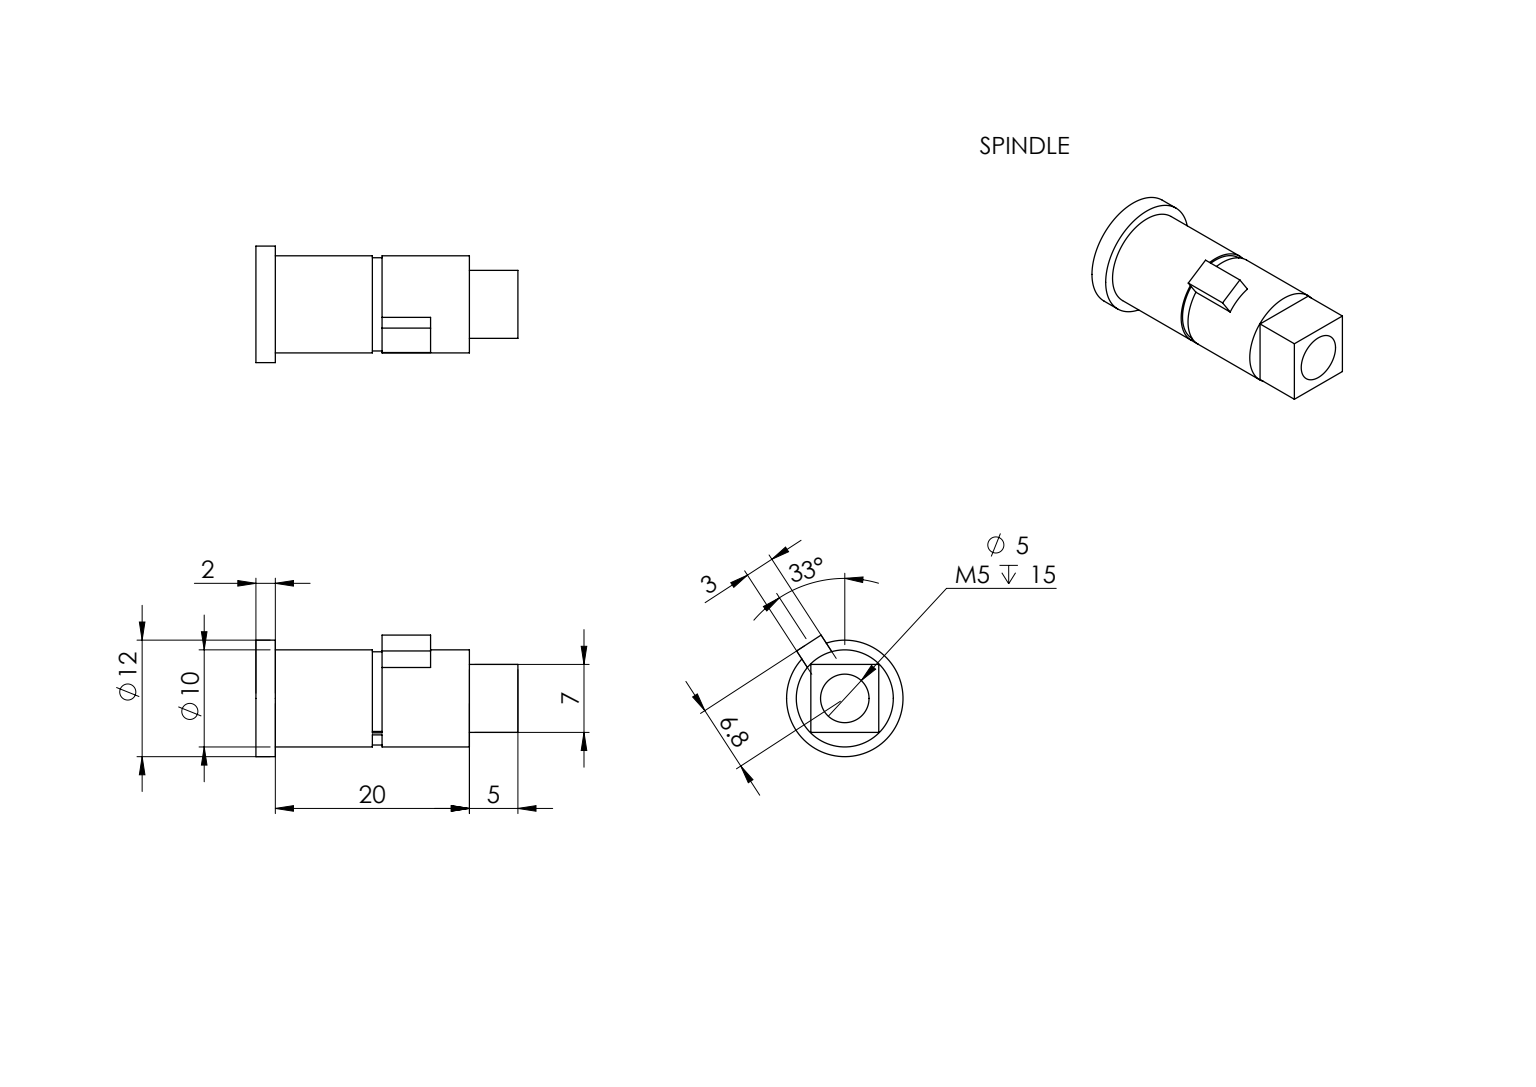
ISO-10303-21;
HEADER;
FILE_DESCRIPTION (('STEP AP214'),
    '1' );
FILE_NAME ('spindle.step',
    '2026-10-27T08:02:39',
    ( '' ),
    ( '' ),
    'SwSTEP 2.0',
    'SolidWorks 2026',
    '' );
FILE_SCHEMA (( 'AUTOMOTIVE_DESIGN' ));
ENDSEC;

DATA;
#32=DIRECTION ( 'NONE',  ( 1.000000000000000000, -0.000000000000000000, 0.000000000000000000 ) ) ;
#36=AXIS2_PLACEMENT_3D ( 'NONE', #6295, #7112, #8236 ) ;
#46=DIRECTION ( 'NONE',  ( 0.000000000000000000, 0.000000000000000000, -1.000000000000000000 ) ) ;
#52=ORIENTED_EDGE ( 'NONE', *, *, #6778, .T. ) ;
#65=DIRECTION ( 'NONE',  ( 0.000000000000000000, 0.6828850436591804574, 0.7305258497456468270 ) ) ;
#79=DIRECTION ( 'NONE',  ( -1.000000000000000000, 0.000000000000000000, 0.000000000000000000 ) ) ;
#82=EDGE_LOOP ( 'NONE', ( #2699, #3221, #1279, #723 ) ) ;
#84=CARTESIAN_POINT ( 'NONE',  ( 36.00000000000000711, -3.606021680338235225, -38.83193945118931367 ) ) ;
#99=DIRECTION ( 'NONE',  ( 0.000000000000000000, 0.6828850436591804574, 0.7305258497456468270 ) ) ;
#101=EDGE_LOOP ( 'NONE', ( #11163, #3779, #6204, #11294 ) ) ;
#116=ORIENTED_EDGE ( 'NONE', *, *, #4223, .F. ) ;
#145=DIRECTION ( 'NONE',  ( 0.000000000000000000, 0.000000000000000000, -1.000000000000000000 ) ) ;
#166=EDGE_LOOP ( 'NONE', ( #4533, #1972 ) ) ;
#181=CYLINDRICAL_SURFACE ( 'NONE', #468, 5.000000000000004441 ) ;
#194=CARTESIAN_POINT ( 'NONE',  ( 51.00000000000000000, -3.499999999999998668, -45.49999999999998579 ) ) ;
#212=CARTESIAN_POINT ( 'NONE',  ( 0.000000000000000000, 0.000000000000000000, 0.000000000000000000 ) ) ;
#214=VERTEX_POINT ( 'NONE', #5344 ) ;
#240=AXIS2_PLACEMENT_3D ( 'NONE', #7909, #5962, #9852 ) ;
#243=CONICAL_SURFACE ( 'NONE', #4238, 2.500000000000002220, 1.029744260000000189 ) ;
#251=LINE ( 'NONE', #9999, #3639 ) ;
#274=AXIS2_PLACEMENT_3D ( 'NONE', #11157, #11099, #1724 ) ;
#281=ORIENTED_EDGE ( 'NONE', *, *, #4388, .F. ) ;
#284=CIRCLE ( 'NONE', #2474, 4.800000000000000711 ) ;
#287=ADVANCED_FACE ( 'NONE', ( #2841 ), #4660, .F. ) ;
#293=PLANE ( 'NONE',  #3827 ) ;
#330=PRODUCT ( 'spindle', 'spindle', '', ( #11158 ) ) ;
#346=ORIENTED_EDGE ( 'NONE', *, *, #9732, .F. ) ;
#349=MANIFOLD_SOLID_BREP ( 'AdvancedHole1', #10962 ) ;
#352=EDGE_CURVE ( 'NONE', #7364, #3914, #3801, .T. ) ;
#364=CARTESIAN_POINT ( 'NONE',  ( 42.00000000000000000, 3.183245106666225510, -38.14423151746819229 ) ) ;
#375=DIRECTION ( 'NONE',  ( 0.000000000000000000, 0.000000000000000000, 1.000000000000000000 ) ) ;
#427=DIRECTION ( 'NONE',  ( 1.000000000000000000, -0.000000000000000000, -0.000000000000000000 ) ) ;
#441=CARTESIAN_POINT ( 'NONE',  ( 46.00000000000000000, 3.500000000000001332, -38.49999999999998579 ) ) ;
#458=CARTESIAN_POINT ( 'NONE',  ( 46.00000000000000000, 6.123233995736773185E-16, -46.99999999999999289 ) ) ;
#468=AXIS2_PLACEMENT_3D ( 'NONE', #2246, #10558, #8702 ) ;
#494=( LENGTH_UNIT ( ) NAMED_UNIT ( * ) SI_UNIT ( .MILLI., .METRE. ) );
#520=DIRECTION ( 'NONE',  ( -1.000000000000000000, -0.000000000000000000, -0.000000000000000000 ) ) ;
#524=ORIENTED_EDGE ( 'NONE', *, *, #1950, .F. ) ;
#553=ORIENTED_EDGE ( 'NONE', *, *, #10197, .F. ) ;
#554=ORIENTED_EDGE ( 'NONE', *, *, #10262, .T. ) ;
#565=ADVANCED_FACE ( 'NONE', ( #4744 ), #6885, .T. ) ;
#574=CARTESIAN_POINT ( 'NONE',  ( 51.00000000000000000, -3.499999999999998668, -38.49999999999998579 ) ) ;
#586=CARTESIAN_POINT ( 'NONE',  ( 42.00000000000000000, 4.817162211711309538, -40.66024322130446222 ) ) ;
#593=EDGE_CURVE ( 'NONE', #6667, #1161, #5812, .T. ) ;
#608=VECTOR ( 'NONE', #3199, 1000.000000000000000 ) ;
#615=AXIS2_PLACEMENT_3D ( 'NONE', #2148, #3107, #7677 ) ;
#627=ORIENTED_EDGE ( 'NONE', *, *, #11894, .F. ) ;
#631=COLOUR_RGB ( '',0.8941176470588234615, 0.8941176470588234615, 0.8941176470588234615 ) ;
#632=AXIS2_PLACEMENT_3D ( 'NONE', #3534, #3664, #4664 ) ;
#638=ADVANCED_FACE ( 'NONE', ( #2934 ), #10626, .T. ) ;
#654=AXIS2_PLACEMENT_3D ( 'NONE', #12142, #12213, #1855 ) ;
#659=PLANE ( 'NONE',  #632 ) ;
#679=ORIENTED_EDGE ( 'NONE', *, *, #2867, .F. ) ;
#681=VERTEX_POINT ( 'NONE', #9507 ) ;
#698=DIRECTION ( 'NONE',  ( 1.000000000000000000, 0.000000000000000000, 0.000000000000000000 ) ) ;
#716=DIRECTION ( 'NONE',  ( -1.000000000000000000, -0.000000000000000000, -0.000000000000000000 ) ) ;
#723=ORIENTED_EDGE ( 'NONE', *, *, #8714, .T. ) ;
#750=DIRECTION ( 'NONE',  ( 0.000000000000000000, 0.000000000000000000, 1.000000000000000000 ) ) ;
#777=VERTEX_POINT ( 'NONE', #5243 ) ;
#787=MECHANICAL_DESIGN_GEOMETRIC_PRESENTATION_REPRESENTATION('',(#4384),#9194);
#812=CARTESIAN_POINT ( 'NONE',  ( 36.00000000000000711, 1.456773409934505593E-31, -36.99999999999998579 ) ) ;
#822=EDGE_CURVE ( 'NONE', #4760, #6667, #10739, .T. ) ;
#832=AXIS2_PLACEMENT_3D ( 'NONE', #4718, #6732, #8723 ) ;
#853=AXIS2_PLACEMENT_3D ( 'NONE', #10883, #7084, #7954 ) ;
#861=AXIS2_PLACEMENT_3D ( 'NONE', #6268, #3378, #6379 ) ;
#863=VERTEX_POINT ( 'NONE', #1425 ) ;
#877=AXIS2_PLACEMENT_3D ( 'NONE', #8794, #2853, #1099 ) ;
#878=SURFACE_STYLE_USAGE ( .BOTH. , #7454 ) ;
#893=DIRECTION ( 'NONE',  ( 0.000000000000000000, 0.000000000000000000, 1.000000000000000000 ) ) ;
#924=ORIENTED_EDGE ( 'NONE', *, *, #6368, .T. ) ;
#951=ADVANCED_FACE ( 'NONE', ( #2674 ), #3495, .T. ) ;
#974=DIRECTION ( 'NONE',  ( 1.000000000000000000, -0.000000000000000000, -0.000000000000000000 ) ) ;
#991=CIRCLE ( 'NONE', #11951, 6.000000000000005329 ) ;
#1006=AXIS2_PLACEMENT_3D ( 'NONE', #1909, #9667, #145 ) ;
#1007=LINE ( 'NONE', #5641, #2212 ) ;
#1068=DIRECTION ( 'NONE',  ( -1.000000000000000000, 0.000000000000000000, 0.000000000000000000 ) ) ;
#1070=CARTESIAN_POINT ( 'NONE',  ( 24.00000000000000000, 0.000000000000000000, -48.00000000000000000 ) ) ;
#1099=DIRECTION ( 'NONE',  ( 0.000000000000000000, 0.000000000000000000, -1.000000000000000000 ) ) ;
#1112=EDGE_CURVE ( 'NONE', #1842, #1155, #6743, .T. ) ;
#1148=DIRECTION ( 'NONE',  ( -1.000000000000000000, -0.000000000000000000, -0.000000000000000000 ) ) ;
#1155=VERTEX_POINT ( 'NONE', #7617 ) ;
#1160=ORIENTED_EDGE ( 'NONE', *, *, #3799, .T. ) ;
#1161=VERTEX_POINT ( 'NONE', #7111 ) ;
#1181=FACE_OUTER_BOUND ( 'NONE', #4103, .T. ) ;
#1196=EDGE_LOOP ( 'NONE', ( #10186, #2981, #11180, #8301 ) ) ;
#1261=CARTESIAN_POINT ( 'NONE',  ( 37.00000000000000711, 1.456773409934505593E-31, -41.99999999999998579 ) ) ;
#1279=ORIENTED_EDGE ( 'NONE', *, *, #11894, .T. ) ;
#1283=ORIENTED_EDGE ( 'NONE', *, *, #11655, .F. ) ;
#1309=CARTESIAN_POINT ( 'NONE',  ( 51.00000000000000000, 0.000000000000000000, -41.99999999999999289 ) ) ;
#1313=DIRECTION ( 'NONE',  ( 0.000000000000000000, 0.000000000000000000, 1.000000000000000000 ) ) ;
#1318=LINE ( 'NONE', #7616, #9969 ) ;
#1362=EDGE_LOOP ( 'NONE', ( #3805, #3426, #3636, #11704 ) ) ;
#1369=DIRECTION ( 'NONE',  ( 1.000000000000000000, -0.000000000000000000, -0.000000000000000000 ) ) ;
#1373=EDGE_LOOP ( 'NONE', ( #11318, #8359, #9664, #4705 ) ) ;
#1425=CARTESIAN_POINT ( 'NONE',  ( 36.00000000000000711, 3.277848209564065307, -38.49347592122088457 ) ) ;
#1438=ORIENTED_EDGE ( 'NONE', *, *, #6782, .T. ) ;
#1457=CIRCLE ( 'NONE', #654, 6.000000000000005329 ) ;
#1472=ORIENTED_EDGE ( 'NONE', *, *, #11211, .F. ) ;
#1480=DIRECTION ( 'NONE',  ( 0.000000000000000000, -0.5446390350150287496, 0.8386705679454229401 ) ) ;
#1481=ORIENTED_EDGE ( 'NONE', *, *, #6301, .T. ) ;
#1513=EDGE_LOOP ( 'NONE', ( #1666, #2104, #8806 ) ) ;
#1525=DIRECTION ( 'NONE',  ( -0.000000000000000000, 0.8386705679454227180, 0.5446390350150290827 ) ) ;
#1533=DIRECTION ( 'NONE',  ( -1.000000000000000000, 0.000000000000000000, 0.000000000000000000 ) ) ;
#1545=ORIENTED_EDGE ( 'NONE', *, *, #3493, .F. ) ;
#1566=ORIENTED_EDGE ( 'NONE', *, *, #6391, .F. ) ;
#1586=AXIS2_PLACEMENT_3D ( 'NONE', #6572, #7575, #9517 ) ;
#1636=DIRECTION ( 'NONE',  ( -1.000000000000000000, 0.000000000000000000, 0.000000000000000000 ) ) ;
#1640=CIRCLE ( 'NONE', #240, 2.500000000000002220 ) ;
#1658=EDGE_CURVE ( 'NONE', #4309, #2267, #8104, .T. ) ;
#1659=AXIS2_PLACEMENT_3D ( 'NONE', #4254, #2260, #4307 ) ;
#1666=ORIENTED_EDGE ( 'NONE', *, *, #1679, .F. ) ;
#1679=EDGE_CURVE ( 'NONE', #11493, #5674, #6035, .T. ) ;
#1698=CARTESIAN_POINT ( 'NONE',  ( 37.00000000000000711, 1.456773409934505593E-31, -41.99999999999998579 ) ) ;
#1711=ORIENTED_EDGE ( 'NONE', *, *, #7878, .F. ) ;
#1712=EDGE_CURVE ( 'NONE', #11907, #4096, #9726, .T. ) ;
#1724=DIRECTION ( 'NONE',  ( 0.000000000000000000, 0.000000000000000000, 1.000000000000000000 ) ) ;
#1750=PRESENTATION_STYLE_ASSIGNMENT (( #878 ) ) ;
#1767=UNCERTAINTY_MEASURE_WITH_UNIT (LENGTH_MEASURE( 1.000000000000000082E-05 ), #3696, 'distance_accuracy_value', 'NONE');
#1792=ORIENTED_EDGE ( 'NONE', *, *, #1712, .F. ) ;
#1814=LINE ( 'NONE', #7453, #11245 ) ;
#1831=DIRECTION ( 'NONE',  ( -1.000000000000000000, 0.000000000000000000, 0.000000000000000000 ) ) ;
#1842=VERTEX_POINT ( 'NONE', #9101 ) ;
#1843=CIRCLE ( 'NONE', #11015, 5.000000000000004441 ) ;
#1855=DIRECTION ( 'NONE',  ( 0.000000000000000000, 0.000000000000000000, 1.000000000000000000 ) ) ;
#1856=ORIENTED_EDGE ( 'NONE', *, *, #3640, .T. ) ;
#1876=ORIENTED_EDGE ( 'NONE', *, *, #6781, .T. ) ;
#1881=CARTESIAN_POINT ( 'NONE',  ( 36.00000000000000000, 0.000000000000000000, -41.99999999999999289 ) ) ;
#1909=CARTESIAN_POINT ( 'NONE',  ( 24.00000000000000000, 0.000000000000000000, -41.99999999999999289 ) ) ;
#1918=ORIENTED_EDGE ( 'NONE', *, *, #4394, .T. ) ;
#1930=FACE_OUTER_BOUND ( 'NONE', #5467, .T. ) ;
#1949=DIRECTION ( 'NONE',  ( -1.000000000000000000, -0.000000000000000000, -0.000000000000000000 ) ) ;
#1950=EDGE_CURVE ( 'NONE', #2088, #863, #7656, .T. ) ;
#1963=ADVANCED_FACE ( 'NONE', ( #7579 ), #5833, .F. ) ;
#1972=ORIENTED_EDGE ( 'NONE', *, *, #352, .F. ) ;
#1987=ORIENTED_EDGE ( 'NONE', *, *, #12032, .T. ) ;
#1998=VECTOR ( 'NONE', #1949, 1000.000000000000000 ) ;
#2005=SURFACE_STYLE_FILL_AREA ( #10559 ) ;
#2011=AXIS2_PLACEMENT_3D ( 'NONE', #4987, #8747, #65 ) ;
#2019=ORIENTED_EDGE ( 'NONE', *, *, #3045, .F. ) ;
#2020=ADVANCED_FACE ( 'NONE', ( #10755 ), #4074, .F. ) ;
#2031=EDGE_CURVE ( 'NONE', #10266, #214, #10881, .T. ) ;
#2036=ORIENTED_EDGE ( 'NONE', *, *, #9936, .T. ) ;
#2046=VECTOR ( 'NONE', #1148, 1000.000000000000000 ) ;
#2067=ADVANCED_FACE ( 'NONE', ( #7767 ), #10646, .F. ) ;
#2068=ORIENTED_EDGE ( 'NONE', *, *, #6778, .F. ) ;
#2075=CIRCLE ( 'NONE', #5670, 6.000000000000005329 ) ;
#2084=DIRECTION ( 'NONE',  ( -1.000000000000000000, 0.000000000000000000, 0.000000000000000000 ) ) ;
#2088=VERTEX_POINT ( 'NONE', #5127 ) ;
#2104=ORIENTED_EDGE ( 'NONE', *, *, #10760, .T. ) ;
#2119=CARTESIAN_POINT ( 'NONE',  ( 46.00000000000000000, 1.456773409934505593E-31, -41.99999999999998579 ) ) ;
#2138=ORIENTED_EDGE ( 'NONE', *, *, #4239, .T. ) ;
#2148=CARTESIAN_POINT ( 'NONE',  ( 37.00000000000000711, 1.456773409934505593E-31, -41.99999999999998579 ) ) ;
#2156=FACE_OUTER_BOUND ( 'NONE', #3853, .T. ) ;
#2168=VECTOR ( 'NONE', #5203, 1000.000000000000000 ) ;
#2185=EDGE_LOOP ( 'NONE', ( #1918, #10168 ) ) ;
#2186=DIRECTION ( 'NONE',  ( 1.000000000000000000, -0.000000000000000000, -0.000000000000000000 ) ) ;
#2191=DIRECTION ( 'NONE',  ( 0.000000000000000000, 0.000000000000000000, -1.000000000000000000 ) ) ;
#2212=VECTOR ( 'NONE', #7517, 1000.000000000000000 ) ;
#2232=( GEOMETRIC_REPRESENTATION_CONTEXT ( 3 ) GLOBAL_UNCERTAINTY_ASSIGNED_CONTEXT ( ( #1767 ) ) GLOBAL_UNIT_ASSIGNED_CONTEXT ( ( #3696, #10502, #2811 ) ) REPRESENTATION_CONTEXT ( 'NONE', 'WORKASPACE' ) );
#2235=PRODUCT_DEFINITION_SHAPE ( 'NONE', 'NONE',  #8707 ) ;
#2246=CARTESIAN_POINT ( 'NONE',  ( 46.00000000000000000, 1.456773409934505593E-31, -41.99999999999998579 ) ) ;
#2258=DIRECTION ( 'NONE',  ( 1.000000000000000000, -0.000000000000000000, 0.000000000000000000 ) ) ;
#2260=DIRECTION ( 'NONE',  ( 1.000000000000000000, 0.000000000000000000, 0.000000000000000000 ) ) ;
#2262=ORIENTED_EDGE ( 'NONE', *, *, #11830, .T. ) ;
#2267=VERTEX_POINT ( 'NONE', #441 ) ;
#2269=PRODUCT_DEFINITION_CONTEXT ( 'detailed design', #4100, 'design' ) ;
#2270=ORIENTED_EDGE ( 'NONE', *, *, #1679, .T. ) ;
#2273=EDGE_CURVE ( 'NONE', #4298, #2396, #12288, .T. ) ;
#2325=LINE ( 'NONE', #5334, #4051 ) ;
#2330=FACE_OUTER_BOUND ( 'NONE', #11963, .T. ) ;
#2331=EDGE_LOOP ( 'NONE', ( #10322, #679, #6415, #5369 ) ) ;
#2341=DIRECTION ( 'NONE',  ( 0.000000000000000000, -0.8386705679454229401, -0.5446390350150287496 ) ) ;
#2345=VERTEX_POINT ( 'NONE', #6804 ) ;
#2350=ORIENTED_EDGE ( 'NONE', *, *, #6782, .F. ) ;
#2367=DIRECTION ( 'NONE',  ( -1.000000000000000000, 0.000000000000000000, 0.000000000000000000 ) ) ;
#2396=VERTEX_POINT ( 'NONE', #9741 ) ;
#2398=VECTOR ( 'NONE', #7063, 1000.000000000000000 ) ;
#2409=AXIS2_PLACEMENT_3D ( 'NONE', #11970, #6359, #3611 ) ;
#2410=ORIENTED_EDGE ( 'NONE', *, *, #6368, .F. ) ;
#2416=CIRCLE ( 'NONE', #10209, 4.800000000000000711 ) ;
#2441=CARTESIAN_POINT ( 'NONE',  ( 36.00000000000000711, 1.456773409934505593E-31, -41.99999999999998579 ) ) ;
#2474=AXIS2_PLACEMENT_3D ( 'NONE', #9604, #32, #99 ) ;
#2496=ADVANCED_FACE ( 'NONE', ( #8170 ), #6110, .T. ) ;
#2500=DIRECTION ( 'NONE',  ( 0.000000000000000000, 0.6828850436591804574, 0.7305258497456468270 ) ) ;
#2511=CARTESIAN_POINT ( 'NONE',  ( 42.00000000000000000, 6.519918414551419517, -39.55446041381592437 ) ) ;
#2518=CARTESIAN_POINT ( 'NONE',  ( 27.38165010660258503, 5.702959862028875726, -38.29645456189778940 ) ) ;
#2535=EDGE_LOOP ( 'NONE', ( #7510, #9842, #2068, #4600 ) ) ;
#2542=FACE_OUTER_BOUND ( 'NONE', #6504, .T. ) ;
#2561=LINE ( 'NONE', #10258, #12006 ) ;
#2588=CARTESIAN_POINT ( 'NONE',  ( 46.00000000000000000, 1.456773409934505593E-31, -41.99999999999998579 ) ) ;
#2593=DIRECTION ( 'NONE',  ( 0.000000000000000000, 0.000000000000000000, 1.000000000000000000 ) ) ;
#2608=FACE_BOUND ( 'NONE', #11084, .T. ) ;
#2636=EDGE_CURVE ( 'NONE', #11907, #8510, #10796, .T. ) ;
#2645=CIRCLE ( 'NONE', #853, 5.000000000000004441 ) ;
#2653=EDGE_CURVE ( 'NONE', #2345, #1161, #6416, .T. ) ;
#2674=FACE_OUTER_BOUND ( 'NONE', #2185, .T. ) ;
#2678=EDGE_LOOP ( 'NONE', ( #3346, #12181, #1566, #116 ) ) ;
#2699=ORIENTED_EDGE ( 'NONE', *, *, #9732, .T. ) ;
#2705=CARTESIAN_POINT ( 'NONE',  ( 51.00000000000000000, 3.061616997868383141E-16, -39.49999999999999289 ) ) ;
#2719=DIRECTION ( 'NONE',  ( 2.598194829928303306E-18, 0.5446390350150290827, -0.8386705679454227180 ) ) ;
#2734=VERTEX_POINT ( 'NONE', #586 ) ;
#2737=DIRECTION ( 'NONE',  ( -0.000000000000000000, 1.000000000000000000, 0.000000000000000000 ) ) ;
#2742=DIRECTION ( 'NONE',  ( 0.000000000000000000, 0.7512545167371323940, -0.6600126143355576902 ) ) ;
#2746=( NAMED_UNIT ( * ) SI_UNIT ( $, .STERADIAN. ) SOLID_ANGLE_UNIT ( ) );
#2773=CARTESIAN_POINT ( 'NONE',  ( 46.00000000000000000, -3.499999999999998668, -38.49999999999998579 ) ) ;
#2811=( NAMED_UNIT ( * ) SI_UNIT ( $, .STERADIAN. ) SOLID_ANGLE_UNIT ( ) );
#2819=EDGE_CURVE ( 'NONE', #11589, #4096, #7431, .T. ) ;
#2822=VECTOR ( 'NONE', #6496, 1000.000000000000000 ) ;
#2841=FACE_OUTER_BOUND ( 'NONE', #4910, .T. ) ;
#2853=DIRECTION ( 'NONE',  ( 1.000000000000000000, 0.000000000000000000, 0.000000000000000000 ) ) ;
#2856=EDGE_LOOP ( 'NONE', ( #3042, #4731, #346, #8495 ) ) ;
#2867=EDGE_CURVE ( 'NONE', #4122, #214, #3911, .T. ) ;
#2901=DIRECTION ( 'NONE',  ( 0.000000000000000000, 0.6828850436591804574, 0.7305258497456468270 ) ) ;
#2932=DIRECTION ( 'NONE',  ( -2.598194829928303306E-18, -0.5446390350150290827, 0.8386705679454227180 ) ) ;
#2934=FACE_OUTER_BOUND ( 'NONE', #7625, .T. ) ;
#2938=ORIENTED_EDGE ( 'NONE', *, *, #4223, .T. ) ;
#2952=DIRECTION ( 'NONE',  ( -1.000000000000000000, 0.000000000000000000, 0.000000000000000000 ) ) ;
#2968=PLANE ( 'NONE',  #877 ) ;
#2979=CARTESIAN_POINT ( 'NONE',  ( 37.00000000000000711, 1.456773409934505593E-31, -41.99999999999998579 ) ) ;
#2981=ORIENTED_EDGE ( 'NONE', *, *, #2031, .F. ) ;
#2984=ORIENTED_EDGE ( 'NONE', *, *, #4535, .T. ) ;
#3042=ORIENTED_EDGE ( 'NONE', *, *, #822, .T. ) ;
#3045=EDGE_CURVE ( 'NONE', #9490, #681, #4090, .T. ) ;
#3086=DIRECTION ( 'NONE',  ( 0.000000000000000000, 0.6828850436591804574, 0.7305258497456468270 ) ) ;
#3107=DIRECTION ( 'NONE',  ( -1.000000000000000000, 0.000000000000000000, 0.000000000000000000 ) ) ;
#3161=SHAPE_DEFINITION_REPRESENTATION ( #2235, #11360 ) ;
#3194=DIRECTION ( 'NONE',  ( 0.000000000000000000, 1.000000000000000000, 0.000000000000000000 ) ) ;
#3199=DIRECTION ( 'NONE',  ( -1.000000000000000000, 0.000000000000000000, 0.000000000000000000 ) ) ;
#3207=EDGE_CURVE ( 'NONE', #2267, #4122, #3466, .T. ) ;
#3215=AXIS2_PLACEMENT_3D ( 'NONE', #9393, #3462, #750 ) ;
#3216=VECTOR ( 'NONE', #6013, 1000.000000000000000 ) ;
#3221=ORIENTED_EDGE ( 'NONE', *, *, #6575, .T. ) ;
#3225=ORIENTED_EDGE ( 'NONE', *, *, #2636, .T. ) ;
#3229=MECHANICAL_DESIGN_GEOMETRIC_PRESENTATION_REPRESENTATION('',(#4626),#7027);
#3243=CONICAL_SURFACE ( 'NONE', #36, 2.500000000000002220, 1.029744260000000189 ) ;
#3277=DIRECTION ( 'NONE',  ( -1.000000000000000000, 0.000000000000000000, 0.000000000000000000 ) ) ;
#3284=ADVANCED_FACE ( 'NONE', ( #5646 ), #9469, .T. ) ;
#3316=DIRECTION ( 'NONE',  ( 0.000000000000000000, 0.000000000000000000, 1.000000000000000000 ) ) ;
#3322=CARTESIAN_POINT ( 'NONE',  ( 37.00000000000000711, 1.456773409934505593E-31, -41.99999999999998579 ) ) ;
#3346=ORIENTED_EDGE ( 'NONE', *, *, #593, .F. ) ;
#3358=CARTESIAN_POINT ( 'NONE',  ( 51.00000000000000000, 3.061616997868380183E-16, -39.49999999999999289 ) ) ;
#3364=ORIENTED_EDGE ( 'NONE', *, *, #6575, .F. ) ;
#3373=CARTESIAN_POINT ( 'NONE',  ( 24.00000000000000000, 0.000000000000000000, -48.00000000000000000 ) ) ;
#3378=DIRECTION ( 'NONE',  ( -1.000000000000000000, 4.770489558936236458E-18, 0.000000000000000000 ) ) ;
#3409=AXIS2_PLACEMENT_3D ( 'NONE', #9944, #7133, #10822 ) ;
#3426=ORIENTED_EDGE ( 'NONE', *, *, #4164, .T. ) ;
#3446=CARTESIAN_POINT ( 'NONE',  ( 46.00000000000000000, 1.456773409934505593E-31, -36.99999999999998579 ) ) ;
#3462=DIRECTION ( 'NONE',  ( -1.000000000000000000, 0.000000000000000000, 0.000000000000000000 ) ) ;
#3466=LINE ( 'NONE', #8401, #7253 ) ;
#3481=DIRECTION ( 'NONE',  ( 0.000000000000000000, 0.000000000000000000, 1.000000000000000000 ) ) ;
#3493=EDGE_CURVE ( 'NONE', #8510, #11907, #2645, .T. ) ;
#3495=PLANE ( 'NONE',  #2409 ) ;
#3534=CARTESIAN_POINT ( 'NONE',  ( 37.00000000000000711, -3.606021680338235225, -38.83193945118931367 ) ) ;
#3536=EDGE_LOOP ( 'NONE', ( #10683, #11862, #1876, #1283 ) ) ;
#3539=CARTESIAN_POINT ( 'NONE',  ( 24.00000000000000000, 0.000000000000000000, -41.99999999999999289 ) ) ;
#3550=CARTESIAN_POINT ( 'NONE',  ( 36.00000000000000000, 0.000000000000000000, -44.50000000000000000 ) ) ;
#3591=AXIS2_PLACEMENT_3D ( 'NONE', #1309, #2186, #8011 ) ;
#3604=CARTESIAN_POINT ( 'NONE',  ( 36.00000000000000711, 1.456773409934505593E-31, -41.99999999999998579 ) ) ;
#3611=DIRECTION ( 'NONE',  ( 0.000000000000000000, 0.000000000000000000, 1.000000000000000000 ) ) ;
#3620=DIRECTION ( 'NONE',  ( -1.000000000000000000, -0.000000000000000000, -0.000000000000000000 ) ) ;
#3636=ORIENTED_EDGE ( 'NONE', *, *, #3045, .T. ) ;
#3639=VECTOR ( 'NONE', #11685, 1000.000000000000000 ) ;
#3640=EDGE_CURVE ( 'NONE', #863, #9490, #8448, .T. ) ;
#3664=DIRECTION ( 'NONE',  ( 0.000000000000000000, 0.6600126143355578012, 0.7512545167371323940 ) ) ;
#3696=( LENGTH_UNIT ( ) NAMED_UNIT ( * ) SI_UNIT ( .MILLI., .METRE. ) );
#3708=CARTESIAN_POINT ( 'NONE',  ( 37.00000000000000711, 1.456773409934505593E-31, -41.99999999999998579 ) ) ;
#3715=EDGE_CURVE ( 'NONE', #6891, #11408, #5460, .T. ) ;
#3779=ORIENTED_EDGE ( 'NONE', *, *, #8048, .T. ) ;
#3787=CARTESIAN_POINT ( 'NONE',  ( 37.00000000000000711, 6.519918414551419517, -39.55446041381592437 ) ) ;
#3793=LINE ( 'NONE', #5795, #8393 ) ;
#3799=EDGE_CURVE ( 'NONE', #7260, #6891, #7703, .T. ) ;
#3801=CIRCLE ( 'NONE', #5994, 5.000000000000004441 ) ;
#3805=ORIENTED_EDGE ( 'NONE', *, *, #12032, .F. ) ;
#3811=AXIS2_PLACEMENT_3D ( 'NONE', #194, #7899, #7952 ) ;
#3813=DIRECTION ( 'NONE',  ( -1.000000000000000000, -0.000000000000000000, -0.000000000000000000 ) ) ;
#3816=AXIS2_PLACEMENT_3D ( 'NONE', #3322, #2258, #3086 ) ;
#3824=ORIENTED_EDGE ( 'NONE', *, *, #3715, .T. ) ;
#3827=AXIS2_PLACEMENT_3D ( 'NONE', #4106, #7928, #11714 ) ;
#3853=EDGE_LOOP ( 'NONE', ( #9207, #6677, #12105, #2036 ) ) ;
#3888=( LENGTH_UNIT ( ) NAMED_UNIT ( * ) SI_UNIT ( .MILLI., .METRE. ) );
#3908=CARTESIAN_POINT ( 'NONE',  ( 36.00000000000000711, -3.277848209564065307, -45.50652407877909411 ) ) ;
#3911=LINE ( 'NONE', #2773, #4430 ) ;
#3914=VERTEX_POINT ( 'NONE', #11546 ) ;
#3931=FACE_OUTER_BOUND ( 'NONE', #1196, .T. ) ;
#3958=ADVANCED_FACE ( 'NONE', ( #12062 ), #10135, .F. ) ;
#4005=CARTESIAN_POINT ( 'NONE',  ( 37.00000000000000711, -3.277848209564066195, -45.50652407877909411 ) ) ;
#4007=VECTOR ( 'NONE', #79, 1000.000000000000000 ) ;
#4009=CARTESIAN_POINT ( 'NONE',  ( 51.00000000000000000, 3.500000000000001332, -38.49999999999998579 ) ) ;
#4035=DIRECTION ( 'NONE',  ( 0.000000000000000000, 0.000000000000000000, 1.000000000000000000 ) ) ;
#4051=VECTOR ( 'NONE', #5279, 1000.000000000000000 ) ;
#4074=CYLINDRICAL_SURFACE ( 'NONE', #11183, 2.500000000000002220 ) ;
#4090=LINE ( 'NONE', #9042, #9251 ) ;
#4096=VERTEX_POINT ( 'NONE', #5629 ) ;
#4100=APPLICATION_CONTEXT ( 'automotive_design' ) ;
#4103=EDGE_LOOP ( 'NONE', ( #6208, #2270, #1481 ) ) ;
#4106=CARTESIAN_POINT ( 'NONE',  ( 51.00000000000000000, -3.499999999999998668, -38.49999999999998579 ) ) ;
#4122=VERTEX_POINT ( 'NONE', #4562 ) ;
#4124=CARTESIAN_POINT ( 'NONE',  ( 36.00000000000000000, 0.000000000000000000, -41.99999999999999289 ) ) ;
#4127=LINE ( 'NONE', #4181, #7391 ) ;
#4130=CARTESIAN_POINT ( 'NONE',  ( 51.00000000000000000, -3.499999999999998668, -45.49999999999998579 ) ) ;
#4164=EDGE_CURVE ( 'NONE', #10334, #9490, #11252, .T. ) ;
#4181=CARTESIAN_POINT ( 'NONE',  ( 51.00000000000000000, -3.499999999999998668, -45.49999999999998579 ) ) ;
#4182=AXIS2_PLACEMENT_3D ( 'NONE', #8957, #2084, #375 ) ;
#4223=EDGE_CURVE ( 'NONE', #1161, #6545, #1814, .T. ) ;
#4228=ORIENTED_EDGE ( 'NONE', *, *, #2653, .F. ) ;
#4238=AXIS2_PLACEMENT_3D ( 'NONE', #4124, #427, #8078 ) ;
#4239=EDGE_CURVE ( 'NONE', #9505, #7260, #10372, .T. ) ;
#4248=ORIENTED_EDGE ( 'NONE', *, *, #352, .T. ) ;
#4254=CARTESIAN_POINT ( 'NONE',  ( 26.00000000000000355, 1.456773409934505593E-31, -41.99999999999998579 ) ) ;
#4273=VERTEX_POINT ( 'NONE', #10744 ) ;
#4298=VERTEX_POINT ( 'NONE', #1070 ) ;
#4307=DIRECTION ( 'NONE',  ( 0.000000000000000000, 0.000000000000000000, -1.000000000000000000 ) ) ;
#4309=VERTEX_POINT ( 'NONE', #9644 ) ;
#4319=ADVANCED_FACE ( 'NONE', ( #8944 ), #181, .T. ) ;
#4330=LINE ( 'NONE', #9689, #9226 ) ;
#4376=EDGE_CURVE ( 'NONE', #8845, #4298, #2075, .T. ) ;
#4384=STYLED_ITEM('',(#12391),#349);
#4388=EDGE_CURVE ( 'NONE', #6632, #7160, #8466, .T. ) ;
#4394=EDGE_CURVE ( 'NONE', #4298, #8845, #11647, .T. ) ;
#4430=VECTOR ( 'NONE', #8538, 1000.000000000000000 ) ;
#4454=ORIENTED_EDGE ( 'NONE', *, *, #9180, .T. ) ;
#4502=CARTESIAN_POINT ( 'NONE',  ( 36.00000000000000711, 1.456773409934505593E-31, -41.99999999999998579 ) ) ;
#4533=ORIENTED_EDGE ( 'NONE', *, *, #10179, .F. ) ;
#4535=EDGE_CURVE ( 'NONE', #11534, #2088, #284, .T. ) ;
#4545=EDGE_LOOP ( 'NONE', ( #11290, #4676, #2938, #9438, #627, #12295, #924, #1160, #4454, #2984, #10958, #1987 ) ) ;
#4546=ADVANCED_FACE ( 'NONE', ( #7734, #11523 ), #2968, .T. ) ;
#4562=CARTESIAN_POINT ( 'NONE',  ( 46.00000000000000000, -3.499999999999998668, -38.49999999999998579 ) ) ;
#4567=DIRECTION ( 'NONE',  ( 0.000000000000000000, 0.6828850436591806794, 0.7305258497456466049 ) ) ;
#4598=DIRECTION ( 'NONE',  ( -1.000000000000000000, 0.000000000000000000, 0.000000000000000000 ) ) ;
#4600=ORIENTED_EDGE ( 'NONE', *, *, #2031, .T. ) ;
#4614=ORIENTED_EDGE ( 'NONE', *, *, #593, .T. ) ;
#4616=CIRCLE ( 'NONE', #3816, 4.800000000000000711 ) ;
#4626=STYLED_ITEM ( 'NONE', ( #1750 ), #7062 ) ;
#4631=DIRECTION ( 'NONE',  ( 1.000000000000000000, -0.000000000000000000, 0.000000000000000000 ) ) ;
#4660=PLANE ( 'NONE',  #4989 ) ;
#4664=DIRECTION ( 'NONE',  ( 0.000000000000000000, 0.7512545167371323940, -0.6600126143355578012 ) ) ;
#4675=ORIENTED_EDGE ( 'NONE', *, *, #1658, .T. ) ;
#4676=ORIENTED_EDGE ( 'NONE', *, *, #2653, .T. ) ;
#4694=DIRECTION ( 'NONE',  ( -1.000000000000000000, -0.000000000000000000, -0.000000000000000000 ) ) ;
#4698=CYLINDRICAL_SURFACE ( 'NONE', #1586, 4.800000000000000711 ) ;
#4705=ORIENTED_EDGE ( 'NONE', *, *, #12169, .T. ) ;
#4717=LINE ( 'NONE', #12083, #7038 ) ;
#4718=CARTESIAN_POINT ( 'NONE',  ( 37.00000000000000711, 1.456773409934505593E-31, -41.99999999999998579 ) ) ;
#4731=ORIENTED_EDGE ( 'NONE', *, *, #8882, .T. ) ;
#4733=CARTESIAN_POINT ( 'NONE',  ( 27.38165010660258503, 0.8169585525225424583, -43.25800585191812075 ) ) ;
#4735=ORIENTED_EDGE ( 'NONE', *, *, #6391, .T. ) ;
#4741=CARTESIAN_POINT ( 'NONE',  ( 36.00000000000000000, 3.061616997868380183E-16, -39.49999999999999289 ) ) ;
#4744=FACE_OUTER_BOUND ( 'NONE', #11269, .T. ) ;
#4750=( NAMED_UNIT ( * ) PLANE_ANGLE_UNIT ( ) SI_UNIT ( $, .RADIAN. ) );
#4754=CARTESIAN_POINT ( 'NONE',  ( 37.00000000000000711, 4.886001309506331935, -37.03844870997966154 ) ) ;
#4760=VERTEX_POINT ( 'NONE', #9290 ) ;
#4827=CARTESIAN_POINT ( 'NONE',  ( 37.00000000000000711, -3.403685371105885427, -38.61548734756097190 ) ) ;
#4910=EDGE_LOOP ( 'NONE', ( #4675, #8408, #7842, #9900 ) ) ;
#4942=LINE ( 'NONE', #5370, #7987 ) ;
#4987=CARTESIAN_POINT ( 'NONE',  ( 37.00000000000000711, 1.456773409934505593E-31, -41.99999999999998579 ) ) ;
#4989=AXIS2_PLACEMENT_3D ( 'NONE', #10521, #5771, #6668 ) ;
#5012=CARTESIAN_POINT ( 'NONE',  ( 36.00000000000000711, 1.456773409934505593E-31, -41.99999999999998579 ) ) ;
#5040=VECTOR ( 'NONE', #10703, 1000.000000000000000 ) ;
#5081=ORIENTED_EDGE ( 'NONE', *, *, #7927, .F. ) ;
#5083=ADVANCED_FACE ( 'NONE', ( #5197 ), #7849, .F. ) ;
#5085=CARTESIAN_POINT ( 'NONE',  ( 36.00000000000000000, 0.000000000000000000, -41.99999999999999289 ) ) ;
#5127=CARTESIAN_POINT ( 'NONE',  ( 37.00000000000000711, 3.277848209564065307, -38.49347592122088457 ) ) ;
#5133=CARTESIAN_POINT ( 'NONE',  ( 34.49784845693389457, 0.000000000000000000, -41.99999999999999289 ) ) ;
#5195=AXIS2_PLACEMENT_3D ( 'NONE', #2119, #3813, #6753 ) ;
#5197=FACE_OUTER_BOUND ( 'NONE', #9694, .T. ) ;
#5203=DIRECTION ( 'NONE',  ( -0.000000000000000000, -0.000000000000000000, 1.000000000000000000 ) ) ;
#5229=LINE ( 'NONE', #9062, #5849 ) ;
#5243=CARTESIAN_POINT ( 'NONE',  ( 36.00000000000000000, 0.000000000000000000, -44.50000000000000000 ) ) ;
#5248=VECTOR ( 'NONE', #1068, 1000.000000000000000 ) ;
#5279=DIRECTION ( 'NONE',  ( -4.000869187770762975E-18, -0.8386705679454229401, -0.5446390350150287496 ) ) ;
#5303=CARTESIAN_POINT ( 'NONE',  ( 37.00000000000000711, -3.756272583685665190, -38.69993692832219523 ) ) ;
#5334=CARTESIAN_POINT ( 'NONE',  ( 42.00000000000000000, 0.8169585525225424583, -43.25800585191812075 ) ) ;
#5344=CARTESIAN_POINT ( 'NONE',  ( 46.00000000000000000, -3.499999999999998668, -45.49999999999998579 ) ) ;
#5369=ORIENTED_EDGE ( 'NONE', *, *, #1658, .F. ) ;
#5370=CARTESIAN_POINT ( 'NONE',  ( 46.00000000000000000, 6.123233995736773185E-16, -46.99999999999999289 ) ) ;
#5418=CARTESIAN_POINT ( 'NONE',  ( 37.00000000000000711, -3.545505594901966262, -38.47446598704267728 ) ) ;
#5446=VECTOR ( 'NONE', #2742, 1000.000000000000114 ) ;
#5453=DIRECTION ( 'NONE',  ( 1.000000000000000000, -0.000000000000000000, -0.000000000000000000 ) ) ;
#5460=LINE ( 'NONE', #12239, #5248 ) ;
#5467=EDGE_LOOP ( 'NONE', ( #7208, #1438, #4248, #11237 ) ) ;
#5509=ORIENTED_EDGE ( 'NONE', *, *, #2636, .F. ) ;
#5511=CARTESIAN_POINT ( 'NONE',  ( 46.00000000000000000, -3.756272583685664301, -38.69993692832219523 ) ) ;
#5527=ADVANCED_FACE ( 'NONE', ( #2608, #2542 ), #10123, .F. ) ;
#5547=FACE_OUTER_BOUND ( 'NONE', #82, .T. ) ;
#5615=CIRCLE ( 'NONE', #8016, 4.800000000000000711 ) ;
#5629=CARTESIAN_POINT ( 'NONE',  ( 37.00000000000000711, 6.123233995736773185E-16, -46.99999999999999289 ) ) ;
#5641=CARTESIAN_POINT ( 'NONE',  ( 27.38165010660258503, 6.519918414551419517, -39.55446041381592437 ) ) ;
#5646=FACE_OUTER_BOUND ( 'NONE', #7474, .T. ) ;
#5653=EDGE_LOOP ( 'NONE', ( #10778, #10884, #7557, #8678 ) ) ;
#5670=AXIS2_PLACEMENT_3D ( 'NONE', #3539, #4598, #2593 ) ;
#5674=VERTEX_POINT ( 'NONE', #4741 ) ;
#5709=DIRECTION ( 'NONE',  ( 1.000000000000000000, -0.000000000000000000, 0.000000000000000000 ) ) ;
#5732=CARTESIAN_POINT ( 'NONE',  ( 51.00000000000000000, 3.500000000000001332, -38.49999999999998579 ) ) ;
#5746=DIRECTION ( 'NONE',  ( 1.000000000000000000, 0.000000000000000000, 0.000000000000000000 ) ) ;
#5754=VECTOR ( 'NONE', #9782, 1000.000000000000000 ) ;
#5766=UNCERTAINTY_MEASURE_WITH_UNIT (LENGTH_MEASURE( 1.000000000000000082E-05 ), #3888, 'distance_accuracy_value', 'NONE');
#5771=DIRECTION ( 'NONE',  ( 0.000000000000000000, -1.000000000000000000, 0.000000000000000000 ) ) ;
#5790=CIRCLE ( 'NONE', #6581, 5.000000000000004441 ) ;
#5795=CARTESIAN_POINT ( 'NONE',  ( 24.00000000000000000, 7.347880794884122694E-16, -35.99999999999999289 ) ) ;
#5809=CARTESIAN_POINT ( 'NONE',  ( 42.00000000000000000, 5.702959862028875726, -38.29645456189778940 ) ) ;
#5812=LINE ( 'NONE', #11676, #10584 ) ;
#5828=VECTOR ( 'NONE', #5453, 1000.000000000000000 ) ;
#5833=PLANE ( 'NONE',  #11980 ) ;
#5835=DIRECTION ( 'NONE',  ( 0.000000000000000000, 0.6828850436591804574, 0.7305258497456468270 ) ) ;
#5844=AXIS2_PLACEMENT_3D ( 'NONE', #3708, #1831, #5835 ) ;
#5849=VECTOR ( 'NONE', #11849, 1000.000000000000000 ) ;
#5850=CYLINDRICAL_SURFACE ( 'NONE', #1006, 6.000000000000005329 ) ;
#5886=DIRECTION ( 'NONE',  ( -1.000000000000000000, -0.000000000000000000, -0.000000000000000000 ) ) ;
#5907=ORIENTED_EDGE ( 'NONE', *, *, #8827, .F. ) ;
#5920=ORIENTED_EDGE ( 'NONE', *, *, #7865, .T. ) ;
#5924=DIRECTION ( 'NONE',  ( 0.000000000000000000, 0.7512545167371323940, -0.6600126143355576902 ) ) ;
#5962=DIRECTION ( 'NONE',  ( 1.000000000000000000, -0.000000000000000000, -0.000000000000000000 ) ) ;
#5965=DIRECTION ( 'NONE',  ( 0.000000000000000000, -0.7091011189803928527, 0.7051068025914618564 ) ) ;
#5994=AXIS2_PLACEMENT_3D ( 'NONE', #10008, #11865, #10880 ) ;
#6010=EDGE_CURVE ( 'NONE', #214, #4309, #7360, .T. ) ;
#6013=DIRECTION ( 'NONE',  ( -1.000000000000000000, -0.000000000000000000, -0.000000000000000000 ) ) ;
#6035=LINE ( 'NONE', #11649, #6962 ) ;
#6056=AXIS2_PLACEMENT_3D ( 'NONE', #212, #4035, #8864 ) ;
#6097=ORIENTED_EDGE ( 'NONE', *, *, #6781, .F. ) ;
#6103=EDGE_LOOP ( 'NONE', ( #2019, #11159, #11832, #7820, #5081, #10530, #281, #1711 ) ) ;
#6110=PLANE ( 'NONE',  #11390 ) ;
#6118=CARTESIAN_POINT ( 'NONE',  ( 26.00000000000000355, 7.347880794884119736E-16, -35.99999999999999289 ) ) ;
#6126=CYLINDRICAL_SURFACE ( 'NONE', #8584, 6.000000000000005329 ) ;
#6130=CARTESIAN_POINT ( 'NONE',  ( 51.00000000000000000, 0.000000000000000000, -41.99999999999999289 ) ) ;
#6154=VERTEX_POINT ( 'NONE', #3787 ) ;
#6169=ORIENTED_EDGE ( 'NONE', *, *, #1712, .T. ) ;
#6179=EDGE_LOOP ( 'NONE', ( #11167, #9671, #1856, #8320 ) ) ;
#6195=DIRECTION ( 'NONE',  ( 0.000000000000000000, 0.6828850436591804574, 0.7305258497456468270 ) ) ;
#6204=ORIENTED_EDGE ( 'NONE', *, *, #7715, .T. ) ;
#6208=ORIENTED_EDGE ( 'NONE', *, *, #10760, .F. ) ;
#6240=DIRECTION ( 'NONE',  ( 0.000000000000000000, 1.000000000000000000, 0.000000000000000000 ) ) ;
#6268=CARTESIAN_POINT ( 'NONE',  ( 42.00000000000000000, -2.003605614753219590E-16, 0.000000000000000000 ) ) ;
#6276=PLANE ( 'NONE',  #11613 ) ;
#6277=EDGE_CURVE ( 'NONE', #4273, #7263, #1640, .T. ) ;
#6289=AXIS2_PLACEMENT_3D ( 'NONE', #9028, #10192, #10021 ) ;
#6295=CARTESIAN_POINT ( 'NONE',  ( 36.00000000000000000, 0.000000000000000000, -41.99999999999999289 ) ) ;
#6301=EDGE_CURVE ( 'NONE', #5674, #777, #8201, .T. ) ;
#6304=CARTESIAN_POINT ( 'NONE',  ( 46.00000000000000000, -3.499999999999998668, -45.49999999999998579 ) ) ;
#6315=DIRECTION ( 'NONE',  ( -1.000000000000000000, 0.000000000000000000, 0.000000000000000000 ) ) ;
#6359=DIRECTION ( 'NONE',  ( -1.000000000000000000, 0.000000000000000000, 0.000000000000000000 ) ) ;
#6368=EDGE_CURVE ( 'NONE', #4096, #7260, #1843, .T. ) ;
#6379=DIRECTION ( 'NONE',  ( -4.770489558936236458E-18, -1.000000000000000000, 0.000000000000000000 ) ) ;
#6391=EDGE_CURVE ( 'NONE', #6545, #4760, #2561, .T. ) ;
#6401=DIRECTION ( 'NONE',  ( 1.000000000000000000, -0.000000000000000000, -0.000000000000000000 ) ) ;
#6415=ORIENTED_EDGE ( 'NONE', *, *, #3207, .F. ) ;
#6416=CIRCLE ( 'NONE', #8234, 5.000000000000004441 ) ;
#6445=VECTOR ( 'NONE', #4694, 1000.000000000000000 ) ;
#6455=CARTESIAN_POINT ( 'NONE',  ( 37.00000000000000711, 4.817162211711309538, -40.66024322130446222 ) ) ;
#6458=ADVANCED_FACE ( 'NONE', ( #8279 ), #6276, .F. ) ;
#6496=DIRECTION ( 'NONE',  ( -1.000000000000000000, -0.000000000000000000, -0.000000000000000000 ) ) ;
#6500=LINE ( 'NONE', #3550, #8978 ) ;
#6504=EDGE_LOOP ( 'NONE', ( #52, #6589, #7569, #8697 ) ) ;
#6544=ORIENTED_EDGE ( 'NONE', *, *, #10179, .T. ) ;
#6545=VERTEX_POINT ( 'NONE', #4754 ) ;
#6549=DIRECTION ( 'NONE',  ( -1.000000000000000000, -0.000000000000000000, -0.000000000000000000 ) ) ;
#6568=SHAPE_REPRESENTATION_RELATIONSHIP ( 'NONE' , 'NONE' ,  #11360, #7062 ) ;
#6572=CARTESIAN_POINT ( 'NONE',  ( 37.00000000000000711, 1.456773409934505593E-31, -41.99999999999998579 ) ) ;
#6575=EDGE_CURVE ( 'NONE', #2734, #11589, #10565, .T. ) ;
#6581=AXIS2_PLACEMENT_3D ( 'NONE', #5012, #3277, #7771 ) ;
#6587=ORIENTED_EDGE ( 'NONE', *, *, #9515, .T. ) ;
#6589=ORIENTED_EDGE ( 'NONE', *, *, #1112, .T. ) ;
#6622=ADVANCED_FACE ( 'NONE', ( #11444 ), #4698, .T. ) ;
#6632=VERTEX_POINT ( 'NONE', #812 ) ;
#6667=VERTEX_POINT ( 'NONE', #364 ) ;
#6668=DIRECTION ( 'NONE',  ( 0.000000000000000000, -0.000000000000000000, -1.000000000000000000 ) ) ;
#6677=ORIENTED_EDGE ( 'NONE', *, *, #10995, .F. ) ;
#6720=ADVANCED_FACE ( 'NONE', ( #7948 ), #6126, .T. ) ;
#6732=DIRECTION ( 'NONE',  ( -1.000000000000000000, 0.000000000000000000, 0.000000000000000000 ) ) ;
#6743=LINE ( 'NONE', #5732, #9813 ) ;
#6753=DIRECTION ( 'NONE',  ( 0.000000000000000000, 0.000000000000000000, 1.000000000000000000 ) ) ;
#6778=EDGE_CURVE ( 'NONE', #10266, #1842, #4127, .T. ) ;
#6781=EDGE_CURVE ( 'NONE', #7263, #4273, #10171, .T. ) ;
#6782=EDGE_CURVE ( 'NONE', #7160, #7364, #4942, .T. ) ;
#6804=CARTESIAN_POINT ( 'NONE',  ( 37.00000000000000711, 1.456773409934505593E-31, -36.99999999999998579 ) ) ;
#6854=DIRECTION ( 'NONE',  ( 1.000000000000000000, -0.000000000000000000, -0.000000000000000000 ) ) ;
#6885=CYLINDRICAL_SURFACE ( 'NONE', #2011, 4.800000000000000711 ) ;
#6891=VERTEX_POINT ( 'NONE', #10073 ) ;
#6931=ORIENTED_EDGE ( 'NONE', *, *, #6981, .F. ) ;
#6940=ORIENTED_EDGE ( 'NONE', *, *, #11655, .T. ) ;
#6962=VECTOR ( 'NONE', #10713, 999.9999999999998863 ) ;
#6981=EDGE_CURVE ( 'NONE', #8609, #4760, #9444, .T. ) ;
#7027=( GEOMETRIC_REPRESENTATION_CONTEXT ( 3 ) GLOBAL_UNCERTAINTY_ASSIGNED_CONTEXT ( ( #5766 ) ) GLOBAL_UNIT_ASSIGNED_CONTEXT ( ( #3888, #4750, #2746 ) ) REPRESENTATION_CONTEXT ( 'NONE', 'WORKASPACE' ) );
#7028=AXIS2_PLACEMENT_3D ( 'NONE', #4733, #8553, #7620 ) ;
#7035=ADVANCED_FACE ( 'NONE', ( #3931 ), #9632, .F. ) ;
#7038=VECTOR ( 'NONE', #716, 1000.000000000000000 ) ;
#7058=VECTOR ( 'NONE', #8512, 1000.000000000000000 ) ;
#7062=ADVANCED_BREP_SHAPE_REPRESENTATION ( '', ( #349, #6056 ), #2232 ) ;
#7063=DIRECTION ( 'NONE',  ( -4.000869187770762975E-18, -0.8386705679454229401, -0.5446390350150287496 ) ) ;
#7084=DIRECTION ( 'NONE',  ( 1.000000000000000000, 0.000000000000000000, 0.000000000000000000 ) ) ;
#7111=CARTESIAN_POINT ( 'NONE',  ( 37.00000000000000711, 3.183245106666227286, -38.14423151746819229 ) ) ;
#7112=DIRECTION ( 'NONE',  ( 1.000000000000000000, -0.000000000000000000, -0.000000000000000000 ) ) ;
#7133=DIRECTION ( 'NONE',  ( -1.000000000000000000, 4.770489558936236458E-18, 0.000000000000000000 ) ) ;
#7145=ORIENTED_EDGE ( 'NONE', *, *, #8929, .T. ) ;
#7160=VERTEX_POINT ( 'NONE', #10794 ) ;
#7170=VERTEX_POINT ( 'NONE', #6118 ) ;
#7197=DIRECTION ( 'NONE',  ( 1.000000000000000000, -0.000000000000000000, -0.000000000000000000 ) ) ;
#7208=ORIENTED_EDGE ( 'NONE', *, *, #4388, .T. ) ;
#7210=CIRCLE ( 'NONE', #3409, 5.000000000000004441 ) ;
#7241=CARTESIAN_POINT ( 'NONE',  ( 37.00000000000000711, 1.456773409934505593E-31, -41.99999999999998579 ) ) ;
#7253=VECTOR ( 'NONE', #12190, 1000.000000000000000 ) ;
#7260=VERTEX_POINT ( 'NONE', #5303 ) ;
#7263=VERTEX_POINT ( 'NONE', #3358 ) ;
#7355=CARTESIAN_POINT ( 'NONE',  ( 37.00000000000000711, 5.702959862028875726, -38.29645456189778940 ) ) ;
#7360=LINE ( 'NONE', #6304, #11803 ) ;
#7364=VERTEX_POINT ( 'NONE', #8251 ) ;
#7371=ORIENTED_EDGE ( 'NONE', *, *, #12169, .F. ) ;
#7391=VECTOR ( 'NONE', #3194, 1000.000000000000000 ) ;
#7424=DIRECTION ( 'NONE',  ( 0.000000000000000000, 0.000000000000000000, 1.000000000000000000 ) ) ;
#7429=VECTOR ( 'NONE', #46, 1000.000000000000000 ) ;
#7431=CIRCLE ( 'NONE', #832, 5.000000000000004441 ) ;
#7449=CARTESIAN_POINT ( 'NONE',  ( 37.00000000000000711, -3.403685371105885427, -38.61548734756097190 ) ) ;
#7453=CARTESIAN_POINT ( 'NONE',  ( 37.00000000000000711, -0.8169585525225422362, -40.74199414808185793 ) ) ;
#7454=SURFACE_SIDE_STYLE ('',( #2005 ) ) ;
#7471=LINE ( 'NONE', #2705, #11592 ) ;
#7474=EDGE_LOOP ( 'NONE', ( #11222, #11281, #10462, #524 ) ) ;
#7510=ORIENTED_EDGE ( 'NONE', *, *, #6010, .T. ) ;
#7511=ORIENTED_EDGE ( 'NONE', *, *, #10379, .F. ) ;
#7517=DIRECTION ( 'NONE',  ( 1.000000000000000000, 0.000000000000000000, 0.000000000000000000 ) ) ;
#7527=ORIENTED_EDGE ( 'NONE', *, *, #2819, .F. ) ;
#7542=VERTEX_POINT ( 'NONE', #574 ) ;
#7557=ORIENTED_EDGE ( 'NONE', *, *, #3799, .F. ) ;
#7565=CIRCLE ( 'NONE', #8167, 2.500000000000002220 ) ;
#7569=ORIENTED_EDGE ( 'NONE', *, *, #8361, .T. ) ;
#7575=DIRECTION ( 'NONE',  ( -1.000000000000000000, 0.000000000000000000, 0.000000000000000000 ) ) ;
#7579=FACE_OUTER_BOUND ( 'NONE', #1362, .T. ) ;
#7580=LINE ( 'NONE', #4009, #5040 ) ;
#7616=CARTESIAN_POINT ( 'NONE',  ( 36.00000000000000711, -3.606021680338235225, -38.83193945118931367 ) ) ;
#7617=CARTESIAN_POINT ( 'NONE',  ( 51.00000000000000000, 3.500000000000001332, -38.49999999999998579 ) ) ;
#7620=DIRECTION ( 'NONE',  ( 0.000000000000000000, -0.8386705679454229401, -0.5446390350150287496 ) ) ;
#7622=ORIENTED_EDGE ( 'NONE', *, *, #9180, .F. ) ;
#7625=EDGE_LOOP ( 'NONE', ( #5509, #6169, #7527, #3364, #10270, #4614, #4228, #11414 ) ) ;
#7656=LINE ( 'NONE', #11446, #4007 ) ;
#7660=CIRCLE ( 'NONE', #9255, 4.800000000000000711 ) ;
#7673=LINE ( 'NONE', #7728, #2046 ) ;
#7677=DIRECTION ( 'NONE',  ( 0.000000000000000000, 0.6828850436591806794, 0.7305258497456466049 ) ) ;
#7702=DIRECTION ( 'NONE',  ( 0.000000000000000000, 0.000000000000000000, -1.000000000000000000 ) ) ;
#7703=LINE ( 'NONE', #11491, #5446 ) ;
#7715=EDGE_CURVE ( 'NONE', #7170, #2396, #991, .T. ) ;
#7728=CARTESIAN_POINT ( 'NONE',  ( 46.00000000000000000, 1.456773409934505593E-31, -36.99999999999998579 ) ) ;
#7734=FACE_BOUND ( 'NONE', #2331, .T. ) ;
#7749=CARTESIAN_POINT ( 'NONE',  ( 51.00000000000000000, -3.499999999999998668, -38.49999999999998579 ) ) ;
#7767=FACE_OUTER_BOUND ( 'NONE', #2535, .T. ) ;
#7771=DIRECTION ( 'NONE',  ( 0.000000000000000000, 0.000000000000000000, 1.000000000000000000 ) ) ;
#7820=ORIENTED_EDGE ( 'NONE', *, *, #10262, .F. ) ;
#7838=CARTESIAN_POINT ( 'NONE',  ( 24.00000000000000000, 7.347880794884119736E-16, -35.99999999999999289 ) ) ;
#7842=ORIENTED_EDGE ( 'NONE', *, *, #1112, .F. ) ;
#7849=CYLINDRICAL_SURFACE ( 'NONE', #6289, 2.500000000000002220 ) ;
#7865=EDGE_CURVE ( 'NONE', #7160, #9505, #9581, .T. ) ;
#7878=EDGE_CURVE ( 'NONE', #681, #6632, #5790, .T. ) ;
#7880=EDGE_LOOP ( 'NONE', ( #11109, #3225 ) ) ;
#7899=DIRECTION ( 'NONE',  ( 0.000000000000000000, 0.000000000000000000, 1.000000000000000000 ) ) ;
#7909=CARTESIAN_POINT ( 'NONE',  ( 51.00000000000000000, 0.000000000000000000, -41.99999999999999289 ) ) ;
#7927=EDGE_CURVE ( 'NONE', #9505, #11408, #1318, .T. ) ;
#7928=DIRECTION ( 'NONE',  ( 0.000000000000000000, 0.000000000000000000, -1.000000000000000000 ) ) ;
#7948=FACE_OUTER_BOUND ( 'NONE', #1373, .T. ) ;
#7952=DIRECTION ( 'NONE',  ( 1.000000000000000000, 0.000000000000000000, -0.000000000000000000 ) ) ;
#7954=DIRECTION ( 'NONE',  ( 0.000000000000000000, 0.000000000000000000, -1.000000000000000000 ) ) ;
#7971=ORIENTED_EDGE ( 'NONE', *, *, #6277, .F. ) ;
#7987=VECTOR ( 'NONE', #3620, 1000.000000000000000 ) ;
#8011=DIRECTION ( 'NONE',  ( 0.000000000000000000, 0.000000000000000000, -1.000000000000000000 ) ) ;
#8016=AXIS2_PLACEMENT_3D ( 'NONE', #8715, #5709, #2901 ) ;
#8048=EDGE_CURVE ( 'NONE', #8845, #7170, #3793, .T. ) ;
#8078=DIRECTION ( 'NONE',  ( 0.000000000000000000, 0.000000000000000000, -1.000000000000000000 ) ) ;
#8104=LINE ( 'NONE', #10844, #2168 ) ;
#8137=CYLINDRICAL_SURFACE ( 'NONE', #9626, 5.000000000000004441 ) ;
#8149=DIRECTION ( 'NONE',  ( 0.000000000000000000, 0.000000000000000000, 1.000000000000000000 ) ) ;
#8152=ORIENTED_EDGE ( 'NONE', *, *, #12250, .F. ) ;
#8167=AXIS2_PLACEMENT_3D ( 'NONE', #1881, #6854, #7702 ) ;
#8170=FACE_OUTER_BOUND ( 'NONE', #2678, .T. ) ;
#8187=CARTESIAN_POINT ( 'NONE',  ( 51.00000000000000000, 0.000000000000000000, 0.000000000000000000 ) ) ;
#8201=CIRCLE ( 'NONE', #10417, 2.500000000000002220 ) ;
#8234=AXIS2_PLACEMENT_3D ( 'NONE', #7241, #1533, #3481 ) ;
#8236=DIRECTION ( 'NONE',  ( 0.000000000000000000, 0.000000000000000000, -1.000000000000000000 ) ) ;
#8251=CARTESIAN_POINT ( 'NONE',  ( 26.00000000000000355, 6.123233995736773185E-16, -46.99999999999999289 ) ) ;
#8279=FACE_OUTER_BOUND ( 'NONE', #6103, .T. ) ;
#8301=ORIENTED_EDGE ( 'NONE', *, *, #10995, .T. ) ;
#8320=ORIENTED_EDGE ( 'NONE', *, *, #4164, .F. ) ;
#8359=ORIENTED_EDGE ( 'NONE', *, *, #4394, .F. ) ;
#8361=EDGE_CURVE ( 'NONE', #1155, #7542, #12135, .T. ) ;
#8379=DIRECTION ( 'NONE',  ( 1.000000000000000000, -0.000000000000000000, 0.000000000000000000 ) ) ;
#8393=VECTOR ( 'NONE', #974, 1000.000000000000000 ) ;
#8401=CARTESIAN_POINT ( 'NONE',  ( 46.00000000000000000, -3.499999999999998668, -38.49999999999998579 ) ) ;
#8402=VERTEX_POINT ( 'NONE', #3908 ) ;
#8408=ORIENTED_EDGE ( 'NONE', *, *, #9936, .F. ) ;
#8425=DIRECTION ( 'NONE',  ( -1.000000000000000000, 0.000000000000000000, 0.000000000000000000 ) ) ;
#8442=ADVANCED_FACE ( 'NONE', ( #9533 ), #5850, .T. ) ;
#8448=CIRCLE ( 'NONE', #9054, 4.800000000000000711 ) ;
#8455=CIRCLE ( 'NONE', #8856, 5.000000000000004441 ) ;
#8465=DIRECTION ( 'NONE',  ( -0.000000000000000000, -0.7051068025914619675, -0.7091011189803928527 ) ) ;
#8466=CIRCLE ( 'NONE', #8663, 5.000000000000004441 ) ;
#8495=ORIENTED_EDGE ( 'NONE', *, *, #6981, .T. ) ;
#8502=AXIS2_PLACEMENT_3D ( 'NONE', #8187, #6315, #3316 ) ;
#8510=VERTEX_POINT ( 'NONE', #10770 ) ;
#8512=DIRECTION ( 'NONE',  ( -1.000000000000000000, 0.000000000000000000, 0.000000000000000000 ) ) ;
#8538=DIRECTION ( 'NONE',  ( 0.000000000000000000, 0.000000000000000000, -1.000000000000000000 ) ) ;
#8553=DIRECTION ( 'NONE',  ( 0.000000000000000000, -0.5446390350150287496, 0.8386705679454229401 ) ) ;
#8556=ADVANCED_FACE ( 'NONE', ( #9152, #12120 ), #9280, .F. ) ;
#8573=CARTESIAN_POINT ( 'NONE',  ( 46.00000000000000000, -3.545505594901965818, -38.47446598704267728 ) ) ;
#8584=AXIS2_PLACEMENT_3D ( 'NONE', #10878, #8949, #9828 ) ;
#8609=VERTEX_POINT ( 'NONE', #2511 ) ;
#8613=AXIS2_PLACEMENT_3D ( 'NONE', #2588, #10224, #10333 ) ;
#8629=DIRECTION ( 'NONE',  ( 0.000000000000000000, -0.000000000000000000, 1.000000000000000000 ) ) ;
#8663=AXIS2_PLACEMENT_3D ( 'NONE', #3604, #8425, #7424 ) ;
#8670=FACE_OUTER_BOUND ( 'NONE', #4545, .T. ) ;
#8678=ORIENTED_EDGE ( 'NONE', *, *, #4239, .F. ) ;
#8697=ORIENTED_EDGE ( 'NONE', *, *, #9102, .T. ) ;
#8702=DIRECTION ( 'NONE',  ( 0.000000000000000000, 0.000000000000000000, 1.000000000000000000 ) ) ;
#8707=PRODUCT_DEFINITION ( 'UNKNOWN', '', #10434, #2269 ) ;
#8714=EDGE_CURVE ( 'NONE', #6154, #8609, #1007, .T. ) ;
#8715=CARTESIAN_POINT ( 'NONE',  ( 36.00000000000000711, 1.456773409934505593E-31, -41.99999999999998579 ) ) ;
#8723=DIRECTION ( 'NONE',  ( 0.000000000000000000, 0.000000000000000000, 1.000000000000000000 ) ) ;
#8727=PLANE ( 'NONE',  #615 ) ;
#8736=DIRECTION ( 'NONE',  ( 1.000000000000000000, -0.000000000000000000, 0.000000000000000000 ) ) ;
#8747=DIRECTION ( 'NONE',  ( -1.000000000000000000, 0.000000000000000000, 0.000000000000000000 ) ) ;
#8770=EDGE_CURVE ( 'NONE', #2088, #10334, #4616, .T. ) ;
#8794=CARTESIAN_POINT ( 'NONE',  ( 46.00000000000000000, 1.456773409934505593E-31, -41.99999999999998579 ) ) ;
#8806=ORIENTED_EDGE ( 'NONE', *, *, #10379, .T. ) ;
#8827=EDGE_CURVE ( 'NONE', #11534, #8402, #8899, .T. ) ;
#8845=VERTEX_POINT ( 'NONE', #7838 ) ;
#8856=AXIS2_PLACEMENT_3D ( 'NONE', #1261, #2367, #1313 ) ;
#8864=DIRECTION ( 'NONE',  ( 1.000000000000000000, 0.000000000000000000, 0.000000000000000000 ) ) ;
#8870=ADVANCED_FACE ( 'NONE', ( #8670 ), #8727, .T. ) ;
#8882=EDGE_CURVE ( 'NONE', #6667, #2734, #7210, .T. ) ;
#8899=LINE ( 'NONE', #4005, #608 ) ;
#8918=ADVANCED_FACE ( 'NONE', ( #1930 ), #8137, .T. ) ;
#8926=FACE_OUTER_BOUND ( 'NONE', #1513, .T. ) ;
#8929=EDGE_CURVE ( 'NONE', #8510, #2345, #9137, .T. ) ;
#8937=CARTESIAN_POINT ( 'NONE',  ( 42.00000000000000000, -0.8169585525225422362, -40.74199414808185793 ) ) ;
#8944=FACE_OUTER_BOUND ( 'NONE', #12175, .T. ) ;
#8949=DIRECTION ( 'NONE',  ( 1.000000000000000000, -0.000000000000000000, -0.000000000000000000 ) ) ;
#8957=CARTESIAN_POINT ( 'NONE',  ( 36.00000000000000711, 1.456773409934505593E-31, -41.99999999999998579 ) ) ;
#8958=CARTESIAN_POINT ( 'NONE',  ( 37.00000000000000711, -3.277848209564065307, -45.50652407877909411 ) ) ;
#8978=VECTOR ( 'NONE', #10120, 999.9999999999998863 ) ;
#9028=CARTESIAN_POINT ( 'NONE',  ( 51.00000000000000000, 0.000000000000000000, -41.99999999999999289 ) ) ;
#9030=ADVANCED_FACE ( 'NONE', ( #5547 ), #9497, .F. ) ;
#9042=CARTESIAN_POINT ( 'NONE',  ( 36.00000000000000711, -3.403685371105885427, -38.61548734756097190 ) ) ;
#9054=AXIS2_PLACEMENT_3D ( 'NONE', #2441, #8379, #6195 ) ;
#9062=CARTESIAN_POINT ( 'NONE',  ( 37.00000000000000711, -3.403685371105885427, -38.61548734756097190 ) ) ;
#9082=EDGE_LOOP ( 'NONE', ( #7371, #10066 ) ) ;
#9101=CARTESIAN_POINT ( 'NONE',  ( 51.00000000000000000, 3.500000000000001332, -45.49999999999998579 ) ) ;
#9102=EDGE_CURVE ( 'NONE', #7542, #10266, #11475, .T. ) ;
#9135=( NAMED_UNIT ( * ) PLANE_ANGLE_UNIT ( ) SI_UNIT ( $, .RADIAN. ) );
#9137=LINE ( 'NONE', #3446, #2822 ) ;
#9152=FACE_BOUND ( 'NONE', #166, .T. ) ;
#9161=UNCERTAINTY_MEASURE_WITH_UNIT (LENGTH_MEASURE( 1.000000000000000082E-05 ), #494, 'distance_accuracy_value', 'NONE');
#9180=EDGE_CURVE ( 'NONE', #6891, #11534, #2416, .T. ) ;
#9194=( GEOMETRIC_REPRESENTATION_CONTEXT ( 3 ) GLOBAL_UNCERTAINTY_ASSIGNED_CONTEXT ( ( #9161 ) ) GLOBAL_UNIT_ASSIGNED_CONTEXT ( ( #494, #9135, #11985 ) ) REPRESENTATION_CONTEXT ( 'NONE', 'WORKASPACE' ) );
#9207=ORIENTED_EDGE ( 'NONE', *, *, #3207, .T. ) ;
#9220=ADVANCED_FACE ( 'NONE', ( #2156 ), #293, .F. ) ;
#9226=VECTOR ( 'NONE', #520, 1000.000000000000000 ) ;
#9251=VECTOR ( 'NONE', #5965, 1000.000000000000000 ) ;
#9255=AXIS2_PLACEMENT_3D ( 'NONE', #4502, #4631, #2500 ) ;
#9256=VECTOR ( 'NONE', #2719, 1000.000000000000000 ) ;
#9280=PLANE ( 'NONE',  #3215 ) ;
#9290=CARTESIAN_POINT ( 'NONE',  ( 42.00000000000000000, 4.886001309506334600, -37.03844870997966154 ) ) ;
#9314=ADVANCED_FACE ( 'NONE', ( #8926 ), #3243, .F. ) ;
#9347=DIRECTION ( 'NONE',  ( -0.000000000000000000, -1.000000000000000000, -0.000000000000000000 ) ) ;
#9373=ADVANCED_FACE ( 'NONE', ( #11152 ), #659, .F. ) ;
#9393=CARTESIAN_POINT ( 'NONE',  ( 26.00000000000000355, 0.000000000000000000, -41.99999999999999289 ) ) ;
#9438=ORIENTED_EDGE ( 'NONE', *, *, #12250, .T. ) ;
#9443=ORIENTED_EDGE ( 'NONE', *, *, #8714, .F. ) ;
#9444=LINE ( 'NONE', #5809, #10553 ) ;
#9454=EDGE_CURVE ( 'NONE', #1842, #4309, #4717, .T. ) ;
#9465=DIRECTION ( 'NONE',  ( 0.000000000000000000, -0.7091011189803927417, 0.7051068025914618564 ) ) ;
#9469=CYLINDRICAL_SURFACE ( 'NONE', #5844, 4.800000000000000711 ) ;
#9472=CARTESIAN_POINT ( 'NONE',  ( 26.00000000000000355, 0.000000000000000000, -41.99999999999999289 ) ) ;
#9490=VERTEX_POINT ( 'NONE', #11329 ) ;
#9497=PLANE ( 'NONE',  #7028 ) ;
#9505=VERTEX_POINT ( 'NONE', #11651 ) ;
#9507=CARTESIAN_POINT ( 'NONE',  ( 36.00000000000000711, -3.545505594901966262, -38.47446598704267728 ) ) ;
#9512=CARTESIAN_POINT ( 'NONE',  ( 37.00000000000000711, -3.403685371105885427, -38.61548734756097190 ) ) ;
#9515=EDGE_CURVE ( 'NONE', #6632, #3914, #7673, .T. ) ;
#9517=DIRECTION ( 'NONE',  ( 0.000000000000000000, 0.6828850436591804574, 0.7305258497456468270 ) ) ;
#9533=FACE_OUTER_BOUND ( 'NONE', #101, .T. ) ;
#9568=DIRECTION ( 'NONE',  ( 4.000869187770762975E-18, 0.8386705679454229401, 0.5446390350150287496 ) ) ;
#9572=CARTESIAN_POINT ( 'NONE',  ( 46.00000000000000000, 4.817162211711311315, -40.66024322130446222 ) ) ;
#9581=CIRCLE ( 'NONE', #4182, 5.000000000000004441 ) ;
#9590=VECTOR ( 'NONE', #9347, 1000.000000000000000 ) ;
#9604=CARTESIAN_POINT ( 'NONE',  ( 37.00000000000000711, 1.456773409934505593E-31, -41.99999999999998579 ) ) ;
#9618=CARTESIAN_POINT ( 'NONE',  ( 51.00000000000000000, -3.499999999999998668, -38.49999999999998579 ) ) ;
#9626=AXIS2_PLACEMENT_3D ( 'NONE', #10998, #6549, #10295 ) ;
#9632=PLANE ( 'NONE',  #11738 ) ;
#9644=CARTESIAN_POINT ( 'NONE',  ( 46.00000000000000000, 3.500000000000001332, -45.49999999999998579 ) ) ;
#9664=ORIENTED_EDGE ( 'NONE', *, *, #2273, .T. ) ;
#9667=DIRECTION ( 'NONE',  ( 1.000000000000000000, -0.000000000000000000, -0.000000000000000000 ) ) ;
#9671=ORIENTED_EDGE ( 'NONE', *, *, #1950, .T. ) ;
#9672=ORIENTED_EDGE ( 'NONE', *, *, #6277, .T. ) ;
#9689=CARTESIAN_POINT ( 'NONE',  ( 51.00000000000000000, -3.499999999999998668, -38.49999999999998579 ) ) ;
#9694=EDGE_LOOP ( 'NONE', ( #1472, #7511, #6940, #9672 ) ) ;
#9726=LINE ( 'NONE', #458, #5754 ) ;
#9732=EDGE_CURVE ( 'NONE', #8609, #2734, #2325, .T. ) ;
#9741=CARTESIAN_POINT ( 'NONE',  ( 26.00000000000000355, 0.000000000000000000, -48.00000000000000000 ) ) ;
#9782=DIRECTION ( 'NONE',  ( -1.000000000000000000, -0.000000000000000000, -0.000000000000000000 ) ) ;
#9801=DIRECTION ( 'NONE',  ( 0.000000000000000000, 0.6828850436591804574, 0.7305258497456468270 ) ) ;
#9804=VECTOR ( 'NONE', #7197, 1000.000000000000000 ) ;
#9813=VECTOR ( 'NONE', #10539, 1000.000000000000000 ) ;
#9828=DIRECTION ( 'NONE',  ( 0.000000000000000000, 0.000000000000000000, -1.000000000000000000 ) ) ;
#9842=ORIENTED_EDGE ( 'NONE', *, *, #9454, .F. ) ;
#9852=DIRECTION ( 'NONE',  ( 0.000000000000000000, 0.000000000000000000, -1.000000000000000000 ) ) ;
#9900=ORIENTED_EDGE ( 'NONE', *, *, #9454, .T. ) ;
#9924=CARTESIAN_POINT ( 'NONE',  ( 27.38165010660258503, -0.8169585525225422362, -40.74199414808185793 ) ) ;
#9936=EDGE_CURVE ( 'NONE', #1155, #2267, #7580, .T. ) ;
#9944=CARTESIAN_POINT ( 'NONE',  ( 42.00000000000000000, 1.456773409934505593E-31, -41.99999999999998579 ) ) ;
#9969=VECTOR ( 'NONE', #5924, 1000.000000000000114 ) ;
#9999=CARTESIAN_POINT ( 'NONE',  ( 37.00000000000000711, 0.8169585525225424583, -43.25800585191812075 ) ) ;
#10008=CARTESIAN_POINT ( 'NONE',  ( 26.00000000000000355, 1.456773409934505593E-31, -41.99999999999998579 ) ) ;
#10021=DIRECTION ( 'NONE',  ( 0.000000000000000000, 0.000000000000000000, -1.000000000000000000 ) ) ;
#10066=ORIENTED_EDGE ( 'NONE', *, *, #7715, .F. ) ;
#10073=CARTESIAN_POINT ( 'NONE',  ( 37.00000000000000711, -3.606021680338235225, -38.83193945118931367 ) ) ;
#10120=DIRECTION ( 'NONE',  ( 0.5150380737757255245, 0.000000000000000000, -0.8571673013836856869 ) ) ;
#10123=PLANE ( 'NONE',  #8502 ) ;
#10135=PLANE ( 'NONE',  #861 ) ;
#10168=ORIENTED_EDGE ( 'NONE', *, *, #4376, .T. ) ;
#10171=CIRCLE ( 'NONE', #3591, 2.500000000000002220 ) ;
#10179=EDGE_CURVE ( 'NONE', #3914, #7364, #12226, .T. ) ;
#10186=ORIENTED_EDGE ( 'NONE', *, *, #2867, .T. ) ;
#10192=DIRECTION ( 'NONE',  ( 1.000000000000000000, -0.000000000000000000, -0.000000000000000000 ) ) ;
#10197=EDGE_CURVE ( 'NONE', #12260, #2345, #8455, .T. ) ;
#10209=AXIS2_PLACEMENT_3D ( 'NONE', #2979, #8736, #9801 ) ;
#10224=DIRECTION ( 'NONE',  ( 1.000000000000000000, 0.000000000000000000, 0.000000000000000000 ) ) ;
#10249=CARTESIAN_POINT ( 'NONE',  ( 51.00000000000000000, -3.499999999999998668, -45.49999999999998579 ) ) ;
#10258=CARTESIAN_POINT ( 'NONE',  ( 27.38165010660258503, 4.886001309506334600, -37.03844870997966154 ) ) ;
#10262=EDGE_CURVE ( 'NONE', #11408, #8402, #7660, .T. ) ;
#10266=VERTEX_POINT ( 'NONE', #10249 ) ;
#10270=ORIENTED_EDGE ( 'NONE', *, *, #8882, .F. ) ;
#10295=DIRECTION ( 'NONE',  ( 0.000000000000000000, 0.000000000000000000, 1.000000000000000000 ) ) ;
#10322=ORIENTED_EDGE ( 'NONE', *, *, #6010, .F. ) ;
#10333=DIRECTION ( 'NONE',  ( 0.000000000000000000, 0.000000000000000000, -1.000000000000000000 ) ) ;
#10334=VERTEX_POINT ( 'NONE', #7449 ) ;
#10372=LINE ( 'NONE', #5511, #11841 ) ;
#10379=EDGE_CURVE ( 'NONE', #777, #5674, #7565, .T. ) ;
#10417=AXIS2_PLACEMENT_3D ( 'NONE', #5085, #11756, #11880 ) ;
#10434=PRODUCT_DEFINITION_FORMATION_WITH_SPECIFIED_SOURCE ( 'ANY', '', #330, .NOT_KNOWN. ) ;
#10462=ORIENTED_EDGE ( 'NONE', *, *, #11295, .T. ) ;
#10473=LINE ( 'NONE', #7355, #9256 ) ;
#10502=( NAMED_UNIT ( * ) PLANE_ANGLE_UNIT ( ) SI_UNIT ( $, .RADIAN. ) );
#10503=LINE ( 'NONE', #8573, #6445 ) ;
#10521=CARTESIAN_POINT ( 'NONE',  ( 51.00000000000000000, 3.500000000000001332, -38.49999999999998579 ) ) ;
#10530=ORIENTED_EDGE ( 'NONE', *, *, #7865, .F. ) ;
#10539=DIRECTION ( 'NONE',  ( -0.000000000000000000, -0.000000000000000000, 1.000000000000000000 ) ) ;
#10553=VECTOR ( 'NONE', #2932, 1000.000000000000000 ) ;
#10558=DIRECTION ( 'NONE',  ( -1.000000000000000000, -0.000000000000000000, -0.000000000000000000 ) ) ;
#10559=FILL_AREA_STYLE ('',( #11309 ) ) ;
#10565=LINE ( 'NONE', #9572, #1998 ) ;
#10584=VECTOR ( 'NONE', #5886, 1000.000000000000000 ) ;
#10626=CYLINDRICAL_SURFACE ( 'NONE', #5195, 5.000000000000004441 ) ;
#10646=PLANE ( 'NONE',  #3811 ) ;
#10681=PLANE ( 'NONE',  #11399 ) ;
#10683=ORIENTED_EDGE ( 'NONE', *, *, #6301, .F. ) ;
#10703=DIRECTION ( 'NONE',  ( -1.000000000000000000, -0.000000000000000000, -0.000000000000000000 ) ) ;
#10713=DIRECTION ( 'NONE',  ( 0.5150380737757255245, 1.049727191973305394E-16, 0.8571673013836856869 ) ) ;
#10739=LINE ( 'NONE', #8937, #2398 ) ;
#10744=CARTESIAN_POINT ( 'NONE',  ( 51.00000000000000000, 0.000000000000000000, -44.50000000000000000 ) ) ;
#10755=FACE_OUTER_BOUND ( 'NONE', #3536, .T. ) ;
#10760=EDGE_CURVE ( 'NONE', #11493, #777, #6500, .T. ) ;
#10770=CARTESIAN_POINT ( 'NONE',  ( 46.00000000000000000, 1.456773409934505593E-31, -36.99999999999998579 ) ) ;
#10778=ORIENTED_EDGE ( 'NONE', *, *, #7927, .T. ) ;
#10794=CARTESIAN_POINT ( 'NONE',  ( 36.00000000000000711, 6.123233995736773185E-16, -46.99999999999999289 ) ) ;
#10796=CIRCLE ( 'NONE', #8613, 5.000000000000004441 ) ;
#10822=DIRECTION ( 'NONE',  ( 0.000000000000000000, -1.000000000000000000, 0.000000000000000000 ) ) ;
#10844=CARTESIAN_POINT ( 'NONE',  ( 46.00000000000000000, 3.500000000000001332, -38.49999999999998579 ) ) ;
#10878=CARTESIAN_POINT ( 'NONE',  ( 24.00000000000000000, 0.000000000000000000, -41.99999999999999289 ) ) ;
#10880=DIRECTION ( 'NONE',  ( 0.000000000000000000, 0.000000000000000000, -1.000000000000000000 ) ) ;
#10881=LINE ( 'NONE', #4130, #3216 ) ;
#10883=CARTESIAN_POINT ( 'NONE',  ( 46.00000000000000000, 1.456773409934505593E-31, -41.99999999999998579 ) ) ;
#10884=ORIENTED_EDGE ( 'NONE', *, *, #3715, .F. ) ;
#10958=ORIENTED_EDGE ( 'NONE', *, *, #8770, .T. ) ;
#10962=CLOSED_SHELL ( 'NONE', ( #11928, #2020, #3284, #6622, #8442, #638, #8918, #4319, #6720, #951, #8556, #4546, #9373, #1963, #8870, #6458, #565, #9030, #2496, #3958, #11052, #2067, #287, #9220, #7035, #5527, #5083, #9314 ) ) ;
#10995=EDGE_CURVE ( 'NONE', #7542, #4122, #4330, .T. ) ;
#10998=CARTESIAN_POINT ( 'NONE',  ( 46.00000000000000000, 1.456773409934505593E-31, -41.99999999999998579 ) ) ;
#11015=AXIS2_PLACEMENT_3D ( 'NONE', #1698, #11188, #8149 ) ;
#11052=ADVANCED_FACE ( 'NONE', ( #2330 ), #10681, .T. ) ;
#11073=LINE ( 'NONE', #12063, #5828 ) ;
#11084=EDGE_LOOP ( 'NONE', ( #7971, #6097 ) ) ;
#11099=DIRECTION ( 'NONE',  ( -1.000000000000000000, 0.000000000000000000, 0.000000000000000000 ) ) ;
#11109=ORIENTED_EDGE ( 'NONE', *, *, #3493, .T. ) ;
#11116=APPLICATION_CONTEXT ( 'automotive_design' ) ;
#11152=FACE_OUTER_BOUND ( 'NONE', #5653, .T. ) ;
#11157=CARTESIAN_POINT ( 'NONE',  ( 24.00000000000000000, 0.000000000000000000, -41.99999999999999289 ) ) ;
#11158=PRODUCT_CONTEXT ( 'NONE', #11116, 'mechanical' ) ;
#11159=ORIENTED_EDGE ( 'NONE', *, *, #3640, .F. ) ;
#11163=ORIENTED_EDGE ( 'NONE', *, *, #4376, .F. ) ;
#11167=ORIENTED_EDGE ( 'NONE', *, *, #8770, .F. ) ;
#11180=ORIENTED_EDGE ( 'NONE', *, *, #9102, .F. ) ;
#11183=AXIS2_PLACEMENT_3D ( 'NONE', #6130, #1369, #2191 ) ;
#11188=DIRECTION ( 'NONE',  ( -1.000000000000000000, 0.000000000000000000, 0.000000000000000000 ) ) ;
#11211=EDGE_CURVE ( 'NONE', #5674, #7263, #7471, .T. ) ;
#11222=ORIENTED_EDGE ( 'NONE', *, *, #4535, .F. ) ;
#11237=ORIENTED_EDGE ( 'NONE', *, *, #9515, .F. ) ;
#11245=VECTOR ( 'NONE', #9568, 1000.000000000000000 ) ;
#11252=LINE ( 'NONE', #9512, #7058 ) ;
#11269=EDGE_LOOP ( 'NONE', ( #5907, #7622, #3824, #554 ) ) ;
#11281=ORIENTED_EDGE ( 'NONE', *, *, #8827, .T. ) ;
#11290=ORIENTED_EDGE ( 'NONE', *, *, #10197, .T. ) ;
#11294=ORIENTED_EDGE ( 'NONE', *, *, #2273, .F. ) ;
#11295=EDGE_CURVE ( 'NONE', #8402, #863, #5615, .T. ) ;
#11309=FILL_AREA_STYLE_COLOUR ( '', #631 ) ;
#11318=ORIENTED_EDGE ( 'NONE', *, *, #8048, .F. ) ;
#11329=CARTESIAN_POINT ( 'NONE',  ( 36.00000000000000711, -3.403685371105885427, -38.61548734756097190 ) ) ;
#11360=SHAPE_REPRESENTATION ( 'spindle', ( #6056 ), #2232 ) ;
#11390=AXIS2_PLACEMENT_3D ( 'NONE', #9924, #1480, #2341 ) ;
#11399=AXIS2_PLACEMENT_3D ( 'NONE', #2518, #1525, #11889 ) ;
#11408=VERTEX_POINT ( 'NONE', #84 ) ;
#11414=ORIENTED_EDGE ( 'NONE', *, *, #8929, .F. ) ;
#11444=FACE_OUTER_BOUND ( 'NONE', #6179, .T. ) ;
#11446=CARTESIAN_POINT ( 'NONE',  ( 37.00000000000000711, 3.277848209564066639, -38.49347592122088457 ) ) ;
#11475=LINE ( 'NONE', #9618, #7429 ) ;
#11491=CARTESIAN_POINT ( 'NONE',  ( 37.00000000000000711, -3.606021680338235225, -38.83193945118931367 ) ) ;
#11493=VERTEX_POINT ( 'NONE', #5133 ) ;
#11523=FACE_OUTER_BOUND ( 'NONE', #7880, .T. ) ;
#11534=VERTEX_POINT ( 'NONE', #8958 ) ;
#11546=CARTESIAN_POINT ( 'NONE',  ( 26.00000000000000355, 1.456773409934505593E-31, -36.99999999999998579 ) ) ;
#11589=VERTEX_POINT ( 'NONE', #6455 ) ;
#11592=VECTOR ( 'NONE', #6401, 1000.000000000000000 ) ;
#11613=AXIS2_PLACEMENT_3D ( 'NONE', #12119, #1636, #4567 ) ;
#11637=ORIENTED_EDGE ( 'NONE', *, *, #7878, .T. ) ;
#11647=CIRCLE ( 'NONE', #274, 6.000000000000005329 ) ;
#11649=CARTESIAN_POINT ( 'NONE',  ( 36.00000000000000000, 3.061616997868383141E-16, -39.49999999999999289 ) ) ;
#11651=CARTESIAN_POINT ( 'NONE',  ( 36.00000000000000711, -3.756272583685665190, -38.69993692832219523 ) ) ;
#11655=EDGE_CURVE ( 'NONE', #777, #4273, #11073, .T. ) ;
#11676=CARTESIAN_POINT ( 'NONE',  ( 46.00000000000000000, 3.183245106666227286, -38.14423151746819229 ) ) ;
#11685=DIRECTION ( 'NONE',  ( 4.000869187770762975E-18, 0.8386705679454229401, 0.5446390350150287496 ) ) ;
#11704=ORIENTED_EDGE ( 'NONE', *, *, #11830, .F. ) ;
#11714=DIRECTION ( 'NONE',  ( -1.000000000000000000, 0.000000000000000000, -0.000000000000000000 ) ) ;
#11738=AXIS2_PLACEMENT_3D ( 'NONE', #7749, #2737, #8629 ) ;
#11756=DIRECTION ( 'NONE',  ( 1.000000000000000000, -0.000000000000000000, -0.000000000000000000 ) ) ;
#11803=VECTOR ( 'NONE', #6240, 1000.000000000000000 ) ;
#11830=EDGE_CURVE ( 'NONE', #12260, #681, #10503, .T. ) ;
#11832=ORIENTED_EDGE ( 'NONE', *, *, #11295, .F. ) ;
#11841=VECTOR ( 'NONE', #5746, 1000.000000000000000 ) ;
#11849=DIRECTION ( 'NONE',  ( 0.000000000000000000, -0.7091011189803928527, 0.7051068025914618564 ) ) ;
#11860=CARTESIAN_POINT ( 'NONE',  ( 46.00000000000000000, 6.123233995736773185E-16, -46.99999999999999289 ) ) ;
#11862=ORIENTED_EDGE ( 'NONE', *, *, #11211, .T. ) ;
#11865=DIRECTION ( 'NONE',  ( 1.000000000000000000, 0.000000000000000000, 0.000000000000000000 ) ) ;
#11880=DIRECTION ( 'NONE',  ( 0.000000000000000000, 0.000000000000000000, -1.000000000000000000 ) ) ;
#11889=DIRECTION ( 'NONE',  ( 0.000000000000000000, -0.5446390350150290827, 0.8386705679454227180 ) ) ;
#11894=EDGE_CURVE ( 'NONE', #11589, #6154, #251, .T. ) ;
#11907=VERTEX_POINT ( 'NONE', #11860 ) ;
#11928=ADVANCED_FACE ( 'NONE', ( #1181 ), #243, .F. ) ;
#11951=AXIS2_PLACEMENT_3D ( 'NONE', #9472, #2952, #893 ) ;
#11963=EDGE_LOOP ( 'NONE', ( #8152, #4735, #6931, #9443 ) ) ;
#11970=CARTESIAN_POINT ( 'NONE',  ( 24.00000000000000000, 0.000000000000000000, -41.99999999999999289 ) ) ;
#11980=AXIS2_PLACEMENT_3D ( 'NONE', #4827, #8465, #9465 ) ;
#11985=( NAMED_UNIT ( * ) SI_UNIT ( $, .STERADIAN. ) SOLID_ANGLE_UNIT ( ) );
#12006=VECTOR ( 'NONE', #698, 1000.000000000000000 ) ;
#12032=EDGE_CURVE ( 'NONE', #10334, #12260, #5229, .T. ) ;
#12062=FACE_OUTER_BOUND ( 'NONE', #2856, .T. ) ;
#12063=CARTESIAN_POINT ( 'NONE',  ( 51.00000000000000000, 0.000000000000000000, -44.50000000000000000 ) ) ;
#12083=CARTESIAN_POINT ( 'NONE',  ( 51.00000000000000000, 3.500000000000001332, -45.49999999999998579 ) ) ;
#12105=ORIENTED_EDGE ( 'NONE', *, *, #8361, .F. ) ;
#12119=CARTESIAN_POINT ( 'NONE',  ( 36.00000000000000711, 1.456773409934505593E-31, -41.99999999999998579 ) ) ;
#12120=FACE_OUTER_BOUND ( 'NONE', #9082, .T. ) ;
#12135=LINE ( 'NONE', #12269, #9590 ) ;
#12142=CARTESIAN_POINT ( 'NONE',  ( 26.00000000000000355, 0.000000000000000000, -41.99999999999999289 ) ) ;
#12169=EDGE_CURVE ( 'NONE', #2396, #7170, #1457, .T. ) ;
#12175=EDGE_LOOP ( 'NONE', ( #1792, #1545, #7145, #553, #2262, #11637, #6587, #6544, #2350, #5920, #2138, #2410 ) ) ;
#12181=ORIENTED_EDGE ( 'NONE', *, *, #822, .F. ) ;
#12190=DIRECTION ( 'NONE',  ( -0.000000000000000000, -1.000000000000000000, -0.000000000000000000 ) ) ;
#12213=DIRECTION ( 'NONE',  ( -1.000000000000000000, 0.000000000000000000, 0.000000000000000000 ) ) ;
#12226=CIRCLE ( 'NONE', #1659, 5.000000000000004441 ) ;
#12239=CARTESIAN_POINT ( 'NONE',  ( 37.00000000000000711, -3.606021680338235225, -38.83193945118931367 ) ) ;
#12250=EDGE_CURVE ( 'NONE', #6545, #6154, #10473, .T. ) ;
#12260=VERTEX_POINT ( 'NONE', #5418 ) ;
#12269=CARTESIAN_POINT ( 'NONE',  ( 51.00000000000000000, -3.499999999999998668, -38.49999999999998579 ) ) ;
#12288=LINE ( 'NONE', #3373, #9804 ) ;
#12295=ORIENTED_EDGE ( 'NONE', *, *, #2819, .T. ) ;
#12385=COLOUR_RGB('Sky Blue',0.24,0.69,0.87);
#12386=FILL_AREA_STYLE_COLOUR('',#12385);
#12387=FILL_AREA_STYLE('',(#12386));
#12388=SURFACE_STYLE_FILL_AREA(#12387);
#12389=SURFACE_SIDE_STYLE('',(#12388));
#12390=SURFACE_STYLE_USAGE(.BOTH.,#12389);
#12391=PRESENTATION_STYLE_ASSIGNMENT((#12390));
ENDSEC;
END-ISO-10303-21;
